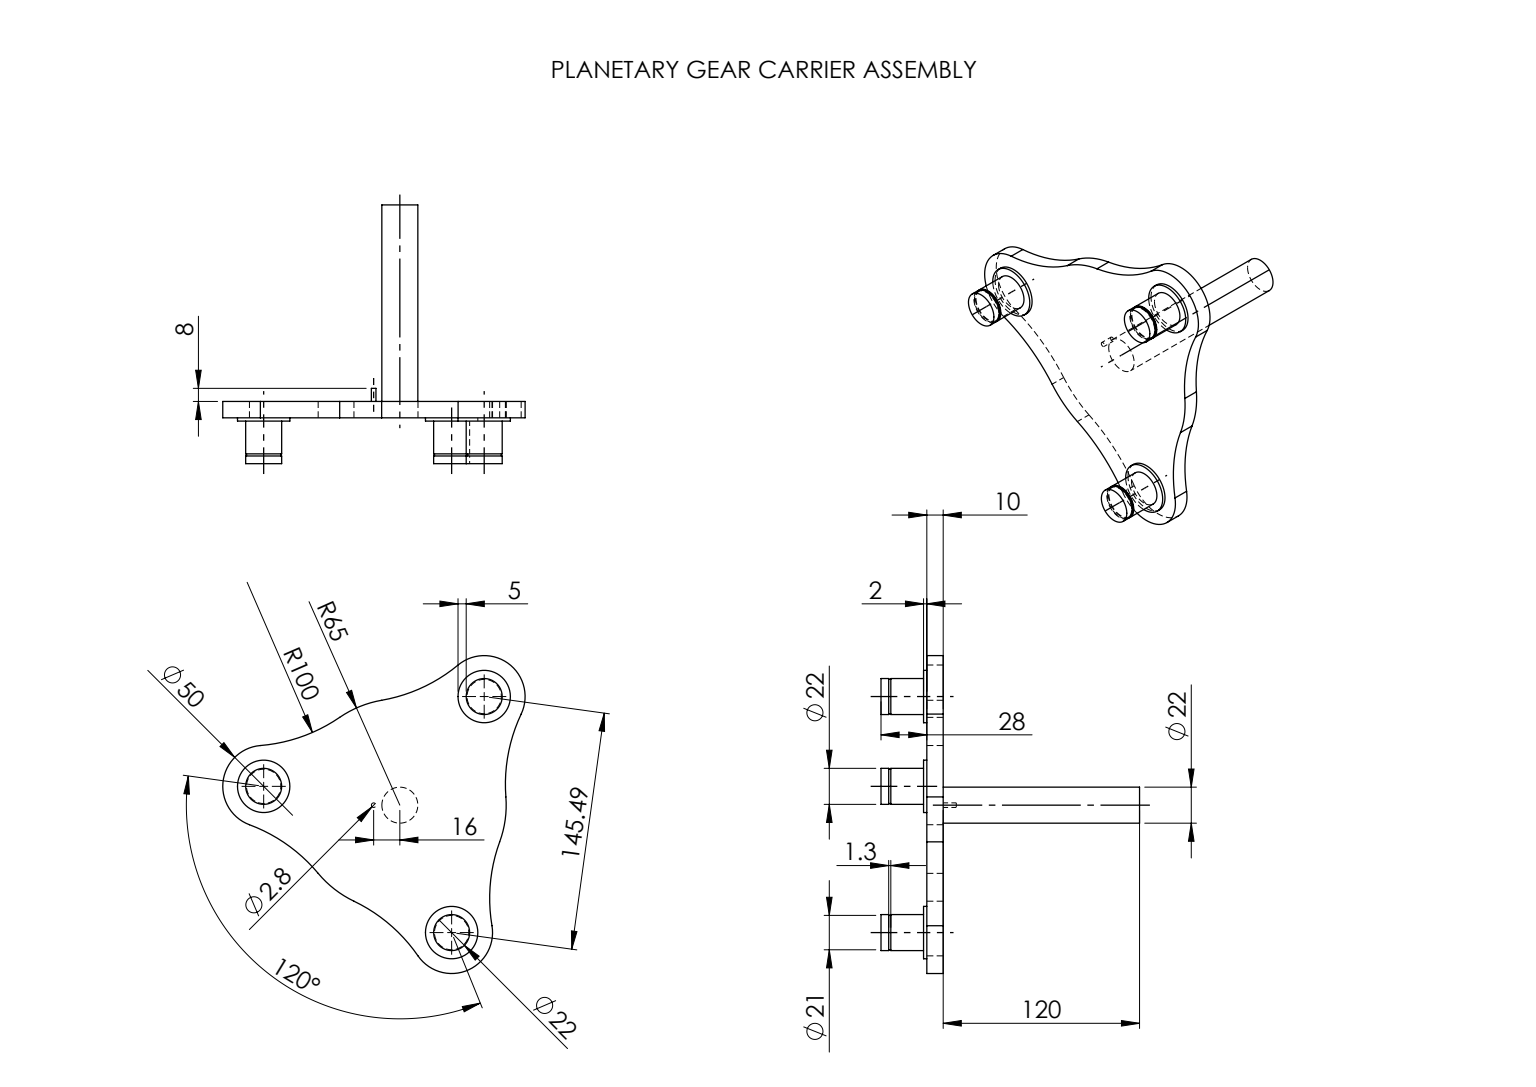
ISO-10303-21;
HEADER;
FILE_DESCRIPTION (('STEP AP214'),
    '1' );
FILE_NAME ('Planetary Gear Carrier Assembly.step',
    '2026-10-08T11:45:07',
    ( '' ),
    ( '' ),
    'SwSTEP 2.0',
    'SolidWorks 2026',
    '' );
FILE_SCHEMA (( 'AUTOMOTIVE_DESIGN' ));
ENDSEC;

DATA;
#3=AXIS2_PLACEMENT_3D ( 'NONE', #17893, #37479, #17456 ) ;
#66=FILL_AREA_STYLE ('',( #17591 ) ) ;
#87=EDGE_CURVE ( 'NONE', #8500, #34172, #3097, .T. ) ;
#134=DIRECTION ( 'NONE',  ( 3.009274222672345096E-17, 1.000000000000000000, -2.455023325076455345E-18 ) ) ;
#185=CARTESIAN_POINT ( 'NONE',  ( 53.30287614962722387, -35.35525454449572180, 69.29271901957299917 ) ) ;
#188=CARTESIAN_POINT ( 'NONE',  ( -36.79328511490363240, -2.055254544495723756, -55.66638716446937707 ) ) ;
#191=EDGE_CURVE ( 'NONE', #37998, #17546, #11534, .T. ) ;
#228=CARTESIAN_POINT ( 'NONE',  ( -102.9608013043458072, -35.35525454449571470, 14.45886780445738218 ) ) ;
#238=FACE_OUTER_BOUND ( 'NONE', #26879, .T. ) ;
#256=MECHANICAL_DESIGN_GEOMETRIC_PRESENTATION_REPRESENTATION('',(#37909),#12862);
#273=AXIS2_PLACEMENT_3D ( 'NONE', #24892, #15283, #24662 ) ;
#300=VERTEX_POINT ( 'NONE', #27299 ) ;
#303=CIRCLE ( 'NONE', #42788, 24.99999999999998934 ) ;
#329=AXIS2_PLACEMENT_3D ( 'NONE', #17951, #33827, #8078 ) ;
#344=EDGE_CURVE ( 'NONE', #2343, #1360, #19212, .T. ) ;
#479=AXIS2_PLACEMENT_3D ( 'NONE', #32329, #9842, #19919 ) ;
#521=SURFACE_STYLE_USAGE ( .BOTH. , #20426 ) ;
#523=ORIENTED_EDGE ( 'NONE', *, *, #10844, .T. ) ;
#530=ORIENTED_EDGE ( 'NONE', *, *, #40112, .T. ) ;
#578=ORIENTED_EDGE ( 'NONE', *, *, #683, .T. ) ;
#610=PLANE ( 'NONE',  #16963 ) ;
#621=CYLINDRICAL_SURFACE ( 'NONE', #22645, 25.00000000000000000 ) ;
#646=DIRECTION ( 'NONE',  ( 1.000000000000000000, -3.009274222672345096E-17, 0.000000000000000000 ) ) ;
#671=DIRECTION ( 'NONE',  ( 3.009274222672345096E-17, 1.000000000000000000, -2.455023325076455345E-18 ) ) ;
#683=EDGE_CURVE ( 'NONE', #23201, #41689, #21250, .T. ) ;
#687=DIRECTION ( 'NONE',  ( -3.009274222672345096E-17, -1.000000000000000000, 2.455023325076454960E-18 ) ) ;
#704=AXIS2_PLACEMENT_3D ( 'NONE', #17398, #27400, #24586 ) ;
#726=SURFACE_STYLE_FILL_AREA ( #66 ) ;
#736=EDGE_CURVE ( 'NONE', #17655, #25229, #13311, .T. ) ;
#775=EDGE_LOOP ( 'NONE', ( #28851, #2876, #36408, #17562 ) ) ;
#804=ADVANCED_FACE ( 'NONE', ( #17457 ), #4302, .T. ) ;
#861=AXIS2_PLACEMENT_3D ( 'NONE', #29019, #9136, #25758 ) ;
#906=ORIENTED_EDGE ( 'NONE', *, *, #34748, .T. ) ;
#938=CARTESIAN_POINT ( 'NONE',  ( 56.05503971749756431, -12.05525454449572464, 8.006123197671259462 ) ) ;
#972=AXIS2_PLACEMENT_3D ( 'NONE', #2544, #29205, #40272 ) ;
#982=EDGE_CURVE ( 'NONE', #41341, #19395, #11317, .T. ) ;
#1003=CARTESIAN_POINT ( 'NONE',  ( 32.30287614962725229, -35.35525454449572180, 69.29271901957299917 ) ) ;
#1019=FILL_AREA_STYLE ('',( #24212 ) ) ;
#1024=DIRECTION ( 'NONE',  ( -1.058513553088275437E-16, -1.000000000000000000, 8.813324511995299047E-17 ) ) ;
#1048=ORIENTED_EDGE ( 'NONE', *, *, #15189, .T. ) ;
#1054=CARTESIAN_POINT ( 'NONE',  ( 26.85238513915532721, -2.055254544495723756, 88.54322126041917329 ) ) ;
#1055=CARTESIAN_POINT ( 'NONE',  ( 42.80287614962790599, -14.05525454449571932, 69.29271901957253021 ) ) ;
#1072=VERTEX_POINT ( 'NONE', #41383 ) ;
#1089=DIRECTION ( 'NONE',  ( 1.000000000000000000, 0.000000000000000000, 0.000000000000000000 ) ) ;
#1168=CYLINDRICAL_SURFACE ( 'NONE', #20654, 11.00000000000023448 ) ;
#1182=CYLINDRICAL_SURFACE ( 'NONE', #32194, 15.99999999999998579 ) ;
#1193=CIRCLE ( 'NONE', #25630, 10.99999999999999822 ) ;
#1295=DIRECTION ( 'NONE',  ( 1.000000000000000000, -3.035766082959412415E-17, 0.000000000000000000 ) ) ;
#1306=ORIENTED_EDGE ( 'NONE', *, *, #9813, .T. ) ;
#1336=CARTESIAN_POINT ( 'NONE',  ( -91.96080130434573618, -35.35525454449571470, 14.45886780445633946 ) ) ;
#1360=VERTEX_POINT ( 'NONE', #26983 ) ;
#1452=DIRECTION ( 'NONE',  ( 3.009274222672345096E-17, 1.000000000000000000, -2.455023325076455345E-18 ) ) ;
#1462=DIRECTION ( 'NONE',  ( 1.000000000000000000, 0.000000000000000000, 0.000000000000000000 ) ) ;
#1493=AXIS2_PLACEMENT_3D ( 'NONE', #14709, #28451, #34754 ) ;
#1543=FACE_BOUND ( 'NONE', #40820, .T. ) ;
#1576=CARTESIAN_POINT ( 'NONE',  ( -91.96080130434580724, -40.05525454449572464, 14.45886780445738218 ) ) ;
#1609=ADVANCED_FACE ( 'NONE', ( #26289 ), #5564, .T. ) ;
#1626=VERTEX_POINT ( 'NONE', #16479 ) ;
#1666=AXIS2_PLACEMENT_3D ( 'NONE', #22494, #18373, #5015 ) ;
#1673=CIRCLE ( 'NONE', #5167, 11.00000000000023803 ) ;
#1684=EDGE_CURVE ( 'NONE', #28176, #33446, #6198, .T. ) ;
#1867=CIRCLE ( 'NONE', #3928, 100.0000000000000711 ) ;
#1931=FACE_OUTER_BOUND ( 'NONE', #23917, .T. ) ;
#1953=CARTESIAN_POINT ( 'NONE',  ( -36.94957890273524725, -12.05525454449572109, 165.5452302238048503 ) ) ;
#1984=ORIENTED_EDGE ( 'NONE', *, *, #344, .T. ) ;
#2031=CARTESIAN_POINT ( 'NONE',  ( 56.25020680251638083, -2.055254544495725977, 2.972870684497274762 ) ) ;
#2040=PLANE ( 'NONE',  #10116 ) ;
#2055=AXIS2_PLACEMENT_3D ( 'NONE', #25182, #17558, #31268 ) ;
#2061=ORIENTED_EDGE ( 'NONE', *, *, #36953, .F. ) ;
#2110=EDGE_LOOP ( 'NONE', ( #9573, #14181, #41848, #41209 ) ) ;
#2116=AXIS2_PLACEMENT_3D ( 'NONE', #27626, #8601, #35009 ) ;
#2146=EDGE_CURVE ( 'NONE', #27084, #7972, #303, .T. ) ;
#2242=EDGE_LOOP ( 'NONE', ( #42171, #17699, #25234, #24047 ) ) ;
#2249=DIRECTION ( 'NONE',  ( -1.000000000000000000, 0.000000000000000000, 0.000000000000000000 ) ) ;
#2261=FACE_OUTER_BOUND ( 'NONE', #9210, .T. ) ;
#2275=DIRECTION ( 'NONE',  ( 1.000000000000000000, 0.000000000000000000, 0.000000000000000000 ) ) ;
#2303=CARTESIAN_POINT ( 'NONE',  ( -19.74979319748359430, -2.055254544495722868, 2.972870684497276539 ) ) ;
#2318=ORIENTED_EDGE ( 'NONE', *, *, #36953, .T. ) ;
#2343=VERTEX_POINT ( 'NONE', #38770 ) ;
#2349=CARTESIAN_POINT ( 'NONE',  ( -8.749793197483594298, -2.055254544495723756, 2.972870684497274762 ) ) ;
#2362=AXIS2_PLACEMENT_3D ( 'NONE', #40085, #9789, #35959 ) ;
#2371=DIRECTION ( 'NONE',  ( 3.009274222672345096E-17, 1.000000000000000000, -2.455023325076454960E-18 ) ) ;
#2386=AXIS2_PLACEMENT_3D ( 'NONE', #30735, #14166, #17017 ) ;
#2406=LINE ( 'NONE', #8773, #18968 ) ;
#2408=PRODUCT_DEFINITION ( 'UNKNOWN', '', #17747, #5868 ) ;
#2428=CIRCLE ( 'NONE', #20624, 11.00000000000023803 ) ;
#2450=ORIENTED_EDGE ( 'NONE', *, *, #18500, .T. ) ;
#2489=ORIENTED_EDGE ( 'NONE', *, *, #34849, .T. ) ;
#2544=CARTESIAN_POINT ( 'NONE',  ( -24.74979319748359785, -2.055254544495722868, 2.972870684497277427 ) ) ;
#2562=CYLINDRICAL_SURFACE ( 'NONE', #12309, 10.99999999999998934 ) ;
#2586=VERTEX_POINT ( 'NONE', #26765 ) ;
#2631=ORIENTED_EDGE ( 'NONE', *, *, #21746, .T. ) ;
#2710=VERTEX_POINT ( 'NONE', #34374 ) ;
#2728=CARTESIAN_POINT ( 'NONE',  ( -80.96080130434580724, -34.05525454449571043, 14.45886780445738395 ) ) ;
#2746=DIRECTION ( 'NONE',  ( -3.009274222672345096E-17, -1.000000000000000000, 2.455023325076455345E-18 ) ) ;
#2762=DIRECTION ( 'NONE',  ( -1.058513553088275437E-16, -1.000000000000000000, 8.813324511995299047E-17 ) ) ;
#2772=EDGE_CURVE ( 'NONE', #25229, #31096, #24877, .T. ) ;
#2872=AXIS2_PLACEMENT_3D ( 'NONE', #31527, #24580, #7523 ) ;
#2876=ORIENTED_EDGE ( 'NONE', *, *, #26728, .T. ) ;
#2898=EDGE_CURVE ( 'NONE', #24559, #19290, #15079, .T. ) ;
#2899=AXIS2_PLACEMENT_3D ( 'NONE', #35121, #37961, #5463 ) ;
#2902=CARTESIAN_POINT ( 'NONE',  ( -80.96080130434580724, -14.05525454449571043, 14.45886780445738395 ) ) ;
#2919=ORIENTED_EDGE ( 'NONE', *, *, #4989, .T. ) ;
#2934=FACE_OUTER_BOUND ( 'NONE', #37750, .T. ) ;
#2987=VERTEX_POINT ( 'NONE', #2902 ) ;
#3055=EDGE_LOOP ( 'NONE', ( #39156, #19434 ) ) ;
#3085=PLANE ( 'NONE',  #20630 ) ;
#3091=VERTEX_POINT ( 'NONE', #36947 ) ;
#3097=CIRCLE ( 'NONE', #15714, 10.99999999999998934 ) ;
#3142=ORIENTED_EDGE ( 'NONE', *, *, #31170, .T. ) ;
#3155=DIRECTION ( 'NONE',  ( -3.009274222672345096E-17, -1.000000000000000000, 2.455023325076454960E-18 ) ) ;
#3191=DIRECTION ( 'NONE',  ( 3.009274222672345096E-17, 1.000000000000000000, -2.455023325076455345E-18 ) ) ;
#3212=FACE_BOUND ( 'NONE', #31827, .T. ) ;
#3262=VECTOR ( 'NONE', #4727, 1000.000000000000000 ) ;
#3286=AXIS2_PLACEMENT_3D ( 'NONE', #23435, #16453, #43031 ) ;
#3299=CIRCLE ( 'NONE', #4699, 11.00000000000023448 ) ;
#3308=APPLICATION_CONTEXT ( 'automotive_design' ) ;
#3319=DIRECTION ( 'NONE',  ( 3.009274222672345096E-17, 1.000000000000000000, -2.455023325076455345E-18 ) ) ;
#3368=ORIENTED_EDGE ( 'NONE', *, *, #14557, .F. ) ;
#3390=AXIS2_PLACEMENT_3D ( 'NONE', #15975, #32107, #19470 ) ;
#3419=CARTESIAN_POINT ( 'NONE',  ( -26.14979319748359643, 5.944745455504278020, 2.972870684497277427 ) ) ;
#3444=( NAMED_UNIT ( * ) SI_UNIT ( $, .STERADIAN. ) SOLID_ANGLE_UNIT ( ) );
#3487=DIRECTION ( 'NONE',  ( -3.009274222672345096E-17, -1.000000000000000000, 2.455023325076454960E-18 ) ) ;
#3534=ORIENTED_EDGE ( 'NONE', *, *, #2146, .F. ) ;
#3555=EDGE_CURVE ( 'NONE', #17655, #26722, #40066, .T. ) ;
#3600=EDGE_CURVE ( 'NONE', #11582, #42604, #23400, .T. ) ;
#3646=DIRECTION ( 'NONE',  ( -1.058513553088275437E-16, -1.000000000000000000, 8.813324511995299047E-17 ) ) ;
#3692=VECTOR ( 'NONE', #37529, 1000.000000000000000 ) ;
#3720=ORIENTED_EDGE ( 'NONE', *, *, #12746, .T. ) ;
#3852=CARTESIAN_POINT ( 'NONE',  ( 0.000000000000000000, 0.000000000000000000, 0.000000000000000000 ) ) ;
#3890=DIRECTION ( 'NONE',  ( -3.009274222672345096E-17, -1.000000000000000000, 2.455023325076454960E-18 ) ) ;
#3898=DIRECTION ( 'NONE',  ( 1.000000000000000000, 0.000000000000000000, 0.000000000000000000 ) ) ;
#3906=EDGE_CURVE ( 'NONE', #6921, #3091, #31737, .T. ) ;
#3928=AXIS2_PLACEMENT_3D ( 'NONE', #1953, #22073, #21653 ) ;
#3933=VECTOR ( 'NONE', #13203, 1000.000000000000000 ) ;
#3936=EDGE_CURVE ( 'NONE', #300, #8500, #22518, .T. ) ;
#3948=VECTOR ( 'NONE', #39099, 1000.000000000000000 ) ;
#3962=ORIENTED_EDGE ( 'NONE', *, *, #5095, .T. ) ;
#3966=AXIS2_PLACEMENT_3D ( 'NONE', #25819, #19275, #32754 ) ;
#3968=CARTESIAN_POINT ( 'NONE',  ( -102.9608013043458072, -40.05525454449572464, 14.45886780445738218 ) ) ;
#4002=DIRECTION ( 'NONE',  ( -1.000000000000000000, 1.084202172485505420E-16, 0.000000000000000000 ) ) ;
#4012=EDGE_CURVE ( 'NONE', #18529, #8193, #11564, .T. ) ;
#4021=ORIENTED_EDGE ( 'NONE', *, *, #14218, .F. ) ;
#4059=LINE ( 'NONE', #24409, #4659 ) ;
#4082=EDGE_CURVE ( 'NONE', #42446, #3091, #42022, .T. ) ;
#4085=DIRECTION ( 'NONE',  ( -1.000000000000000000, 0.000000000000000000, 0.000000000000000000 ) ) ;
#4116=EDGE_CURVE ( 'NONE', #4270, #2710, #25536, .T. ) ;
#4159=EDGE_CURVE ( 'NONE', #19198, #23201, #33152, .T. ) ;
#4169=VERTEX_POINT ( 'NONE', #10441 ) ;
#4257=ORIENTED_EDGE ( 'NONE', *, *, #42315, .F. ) ;
#4270=VERTEX_POINT ( 'NONE', #28654 ) ;
#4278=ORIENTED_EDGE ( 'NONE', *, *, #5722, .F. ) ;
#4293=ADVANCED_FACE ( 'NONE', ( #22133, #38234 ), #15153, .F. ) ;
#4302=CYLINDRICAL_SURFACE ( 'NONE', #2386, 64.99999999999997158 ) ;
#4340=DIRECTION ( 'NONE',  ( -3.009274222672345096E-17, -1.000000000000000000, 2.455023325076455345E-18 ) ) ;
#4359=DIRECTION ( 'NONE',  ( -1.000000000000000000, 0.000000000000000000, 0.000000000000000000 ) ) ;
#4445=ORIENTED_EDGE ( 'NONE', *, *, #23810, .F. ) ;
#4470=SHAPE_REPRESENTATION_RELATIONSHIP ( 'NONE' , 'NONE' ,  #10434, #29166 ) ;
#4495=DIRECTION ( 'NONE',  ( 2.731800627175558911E-17, 1.000000000000000000, -3.170996607629411740E-18 ) ) ;
#4504=AXIS2_PLACEMENT_3D ( 'NONE', #32846, #33283, #16286 ) ;
#4510=DIRECTION ( 'NONE',  ( -3.009274222672345712E-17, -1.000000000000000000, 2.455023325076455345E-18 ) ) ;
#4512=( NAMED_UNIT ( * ) SI_UNIT ( $, .STERADIAN. ) SOLID_ANGLE_UNIT ( ) );
#4543=AXIS2_PLACEMENT_3D ( 'NONE', #43182, #14019, #36672 ) ;
#4544=DIRECTION ( 'NONE',  ( -3.009274222672345096E-17, -1.000000000000000000, 2.455023325076455345E-18 ) ) ;
#4546=CARTESIAN_POINT ( 'NONE',  ( 42.80287614962796994, -2.055254544495723756, 69.29271901957280022 ) ) ;
#4608=CYLINDRICAL_SURFACE ( 'NONE', #15601, 10.49999999999999467 ) ;
#4618=DIRECTION ( 'NONE',  ( 1.000000000000000000, -3.469446951953615421E-17, 0.000000000000000000 ) ) ;
#4644=CIRCLE ( 'NONE', #25586, 100.0000000000000000 ) ;
#4645=DIRECTION ( 'NONE',  ( -1.000000000000000000, 1.084202172485505420E-16, 0.000000000000000000 ) ) ;
#4655=ORIENTED_EDGE ( 'NONE', *, *, #2898, .F. ) ;
#4659=VECTOR ( 'NONE', #14353, 1000.000000000000000 ) ;
#4675=FACE_OUTER_BOUND ( 'NONE', #35556, .T. ) ;
#4688=AXIS2_PLACEMENT_3D ( 'NONE', #26736, #23915, #36969 ) ;
#4699=AXIS2_PLACEMENT_3D ( 'NONE', #10313, #23225, #7236 ) ;
#4705=VERTEX_POINT ( 'NONE', #9098 ) ;
#4727=DIRECTION ( 'NONE',  ( -3.009274222672345096E-17, -1.000000000000000000, 2.455023325076454960E-18 ) ) ;
#4785=DIRECTION ( 'NONE',  ( 1.000000000000000000, -3.469446951953611107E-17, 0.000000000000000000 ) ) ;
#4826=DIRECTION ( 'NONE',  ( 1.058513553088275437E-16, 1.000000000000000000, -8.813324511995299047E-17 ) ) ;
#4836=DIRECTION ( 'NONE',  ( -1.000000000000000000, 0.000000000000000000, 0.000000000000000000 ) ) ;
#4847=CARTESIAN_POINT ( 'NONE',  ( -102.0670434220619427, -12.05525454449572109, 139.0496534599708980 ) ) ;
#4960=CIRCLE ( 'NONE', #11235, 24.99999999999998934 ) ;
#4967=ORIENTED_EDGE ( 'NONE', *, *, #5545, .T. ) ;
#4989=EDGE_CURVE ( 'NONE', #41689, #18808, #4960, .T. ) ;
#5015=DIRECTION ( 'NONE',  ( -1.000000000000000000, 2.668805347656627603E-17, 0.000000000000000000 ) ) ;
#5023=VECTOR ( 'NONE', #21662, 1000.000000000000000 ) ;
#5026=CYLINDRICAL_SURFACE ( 'NONE', #2899, 16.00000000000023448 ) ;
#5037=DIRECTION ( 'NONE',  ( -1.000000000000000000, 0.000000000000000000, 0.000000000000000000 ) ) ;
#5072=CARTESIAN_POINT ( 'NONE',  ( 22.90854556226730310, -35.35525454449573601, -74.83297477053802993 ) ) ;
#5094=DIRECTION ( 'NONE',  ( -1.000000000000000000, 0.000000000000000000, 0.000000000000000000 ) ) ;
#5095=EDGE_CURVE ( 'NONE', #42446, #30653, #33512, .T. ) ;
#5101=FACE_BOUND ( 'NONE', #19325, .T. ) ;
#5115=ADVANCED_FACE ( 'NONE', ( #2261 ), #42190, .F. ) ;
#5143=DIRECTION ( 'NONE',  ( -3.009274222672345096E-17, -1.000000000000000000, 2.455023325076455345E-18 ) ) ;
#5150=VERTEX_POINT ( 'NONE', #12349 ) ;
#5154=DIRECTION ( 'NONE',  ( -1.000000000000000000, 1.577021341797098793E-16, 0.000000000000000000 ) ) ;
#5165=LINE ( 'NONE', #38531, #21399 ) ;
#5167=AXIS2_PLACEMENT_3D ( 'NONE', #12668, #42725, #6310 ) ;
#5180=DIRECTION ( 'NONE',  ( -3.009274222672345096E-17, -1.000000000000000000, 2.455023325076454960E-18 ) ) ;
#5185=ADVANCED_FACE ( 'NONE', ( #19547 ), #39339, .F. ) ;
#5193=DIRECTION ( 'NONE',  ( 1.000000000000000000, -3.469446951953614189E-17, 0.000000000000000000 ) ) ;
#5255=VECTOR ( 'NONE', #29258, 1000.000000000000000 ) ;
#5327=DIRECTION ( 'NONE',  ( 1.000000000000000000, 0.000000000000000000, 0.000000000000000000 ) ) ;
#5343=CYLINDRICAL_SURFACE ( 'NONE', #5646, 10.99999999999999645 ) ;
#5371=DIRECTION ( 'NONE',  ( -1.058513553088275437E-16, -1.000000000000000000, 8.813324511995299047E-17 ) ) ;
#5388=DIRECTION ( 'NONE',  ( -1.058513553088275437E-16, -1.000000000000000000, 8.813324511995299047E-17 ) ) ;
#5394=AXIS2_PLACEMENT_3D ( 'NONE', #15186, #24574, #5327 ) ;
#5397=DIRECTION ( 'NONE',  ( 3.009274222672345096E-17, 1.000000000000000000, -2.455023325076454960E-18 ) ) ;
#5441=ORIENTED_EDGE ( 'NONE', *, *, #32084, .T. ) ;
#5463=DIRECTION ( 'NONE',  ( 1.000000000000000000, 0.000000000000000000, 0.000000000000000000 ) ) ;
#5482=DIRECTION ( 'NONE',  ( 2.932542530036133930E-17, 1.000000000000000000, -5.216001792149171863E-18 ) ) ;
#5515=LINE ( 'NONE', #25199, #25032 ) ;
#5545=EDGE_CURVE ( 'NONE', #28510, #24559, #28465, .T. ) ;
#5564=CYLINDRICAL_SURFACE ( 'NONE', #32515, 15.99999999999999289 ) ;
#5601=EDGE_CURVE ( 'NONE', #23828, #27222, #5515, .T. ) ;
#5624=EDGE_CURVE ( 'NONE', #8001, #13563, #38204, .T. ) ;
#5627=DIRECTION ( 'NONE',  ( -1.000000000000000000, 1.058513553088275437E-16, 0.000000000000000000 ) ) ;
#5646=AXIS2_PLACEMENT_3D ( 'NONE', #9686, #36068, #2249 ) ;
#5684=CARTESIAN_POINT ( 'NONE',  ( 22.90854556226710415, -14.05525454449572997, -74.83297477053821467 ) ) ;
#5695=ORIENTED_EDGE ( 'NONE', *, *, #8889, .T. ) ;
#5722=EDGE_CURVE ( 'NONE', #11152, #9805, #41632, .T. ) ;
#5760=CIRCLE ( 'NONE', #38489, 10.49999999999998934 ) ;
#5768=DIRECTION ( 'NONE',  ( 1.000000000000000000, -3.035766082959414264E-17, 0.000000000000000000 ) ) ;
#5807=ADVANCED_FACE ( 'NONE', ( #28179 ), #11597, .T. ) ;
#5867=CARTESIAN_POINT ( 'NONE',  ( -58.65872368235312706, -2.055254544495720648, -38.66963954070958209 ) ) ;
#5868=PRODUCT_DEFINITION_CONTEXT ( 'detailed design', #3308, 'design' ) ;
#5879=CARTESIAN_POINT ( 'NONE',  ( -24.74979319748359785, 5.944745455504278020, 2.972870684497277427 ) ) ;
#5949=CARTESIAN_POINT ( 'NONE',  ( 56.25020680251638083, -12.05525454449572642, 2.972870684497274762 ) ) ;
#5968=ORIENTED_EDGE ( 'NONE', *, *, #21175, .T. ) ;
#6015=ORIENTED_EDGE ( 'NONE', *, *, #42762, .T. ) ;
#6031=EDGE_LOOP ( 'NONE', ( #27869, #35477, #16575, #38468 ) ) ;
#6088=PLANE ( 'NONE',  #31849 ) ;
#6133=DIRECTION ( 'NONE',  ( -3.009274222672345096E-17, -1.000000000000000000, 2.455023325076454960E-18 ) ) ;
#6160=EDGE_CURVE ( 'NONE', #39731, #1072, #21699, .T. ) ;
#6198=LINE ( 'NONE', #19544, #3933 ) ;
#6277=ORIENTED_EDGE ( 'NONE', *, *, #37983, .F. ) ;
#6283=VERTEX_POINT ( 'NONE', #29904 ) ;
#6301=CARTESIAN_POINT ( 'NONE',  ( -91.96080130434580724, -40.05525454449572464, 14.45886780445738218 ) ) ;
#6310=DIRECTION ( 'NONE',  ( 1.000000000000000000, 0.000000000000000000, 0.000000000000000000 ) ) ;
#6352=CIRCLE ( 'NONE', #40476, 15.99999999999998934 ) ;
#6357=DIRECTION ( 'NONE',  ( 1.000000000000000000, -3.469446951953614189E-17, 0.000000000000000000 ) ) ;
#6360=AXIS2_PLACEMENT_3D ( 'NONE', #6405, #12555, #16478 ) ;
#6391=ORIENTED_EDGE ( 'NONE', *, *, #24742, .T. ) ;
#6401=CYLINDRICAL_SURFACE ( 'NONE', #9809, 10.49999999999998934 ) ;
#6402=PRODUCT_DEFINITION_SHAPE ( 'NONE', 'NONE',  #2408 ) ;
#6405=CARTESIAN_POINT ( 'NONE',  ( 22.90854556226722138, -12.05525454449572464, -74.83297477053847047 ) ) ;
#6457=EDGE_LOOP ( 'NONE', ( #24731, #2631, #43148, #11821 ) ) ;
#6465=DIRECTION ( 'NONE',  ( -3.009274222672345096E-17, -1.000000000000000000, 2.455023325076454960E-18 ) ) ;
#6547=ORIENTED_EDGE ( 'NONE', *, *, #5722, .T. ) ;
#6551=ADVANCED_FACE ( 'NONE', ( #12140 ), #32616, .T. ) ;
#6555=ORIENTED_EDGE ( 'NONE', *, *, #4116, .T. ) ;
#6577=AXIS2_PLACEMENT_3D ( 'NONE', #7725, #18042, #31079 ) ;
#6596=ORIENTED_EDGE ( 'NONE', *, *, #42956, .T. ) ;
#6600=LINE ( 'NONE', #3968, #32014 ) ;
#6606=EDGE_CURVE ( 'NONE', #2710, #4270, #13019, .T. ) ;
#6610=ORIENTED_EDGE ( 'NONE', *, *, #2772, .F. ) ;
#6629=DIRECTION ( 'NONE',  ( -1.000000000000000000, 3.469446951953614189E-17, 0.000000000000000000 ) ) ;
#6683=EDGE_CURVE ( 'NONE', #12272, #25229, #4644, .T. ) ;
#6692=ORIENTED_EDGE ( 'NONE', *, *, #15852, .F. ) ;
#6712=CIRCLE ( 'NONE', #19996, 10.99999999999998934 ) ;
#6714=CARTESIAN_POINT ( 'NONE',  ( -75.96080130434582145, -12.05525454449571043, 14.45886780445738218 ) ) ;
#6727=DIRECTION ( 'NONE',  ( 3.009274222672345096E-17, 1.000000000000000000, -2.455023325076454960E-18 ) ) ;
#6813=LINE ( 'NONE', #15802, #29424 ) ;
#6816=VERTEX_POINT ( 'NONE', #11016 ) ;
#6832=DIRECTION ( 'NONE',  ( -1.000000000000000000, 0.000000000000000000, 0.000000000000000000 ) ) ;
#6853=DIRECTION ( 'NONE',  ( -1.000000000000000000, 0.000000000000000000, 0.000000000000000000 ) ) ;
#6885=DIRECTION ( 'NONE',  ( -3.009274222672345096E-17, -1.000000000000000000, 2.455023325076454960E-18 ) ) ;
#6891=ORIENTED_EDGE ( 'NONE', *, *, #6606, .F. ) ;
#6921=VERTEX_POINT ( 'NONE', #15378 ) ;
#6935=ORIENTED_EDGE ( 'NONE', *, *, #39888, .F. ) ;
#6954=DIRECTION ( 'NONE',  ( 3.009274222672345096E-17, 1.000000000000000000, -2.455023325076454960E-18 ) ) ;
#6974=CIRCLE ( 'NONE', #20263, 10.49999999999999467 ) ;
#6978=DIRECTION ( 'NONE',  ( 3.009274222672345096E-17, 1.000000000000000000, -2.455023325076454960E-18 ) ) ;
#7027=FACE_OUTER_BOUND ( 'NONE', #6031, .T. ) ;
#7080=EDGE_CURVE ( 'NONE', #5150, #12532, #36252, .T. ) ;
#7091=FACE_OUTER_BOUND ( 'NONE', #16629, .T. ) ;
#7103=EDGE_CURVE ( 'NONE', #4270, #4705, #13587, .T. ) ;
#7107=ORIENTED_EDGE ( 'NONE', *, *, #32284, .T. ) ;
#7116=CARTESIAN_POINT ( 'NONE',  ( 146.1418929693599580, -2.055254544495727309, -53.89157828313137344 ) ) ;
#7144=EDGE_LOOP ( 'NONE', ( #16694, #32181 ) ) ;
#7149=CARTESIAN_POINT ( 'NONE',  ( 42.80287614962790599, -34.05525454449571754, 69.29271901957253021 ) ) ;
#7179=CARTESIAN_POINT ( 'NONE',  ( 52.26814377733353467, -2.055254544495723756, -19.42827587850796434 ) ) ;
#7215=AXIS2_PLACEMENT_3D ( 'NONE', #14897, #31025, #14684 ) ;
#7236=DIRECTION ( 'NONE',  ( -1.000000000000000000, 1.577021341797063787E-16, 0.000000000000000000 ) ) ;
#7237=CIRCLE ( 'NONE', #36504, 10.99999999999998934 ) ;
#7242=ORIENTED_EDGE ( 'NONE', *, *, #3906, .F. ) ;
#7394=AXIS2_PLACEMENT_3D ( 'NONE', #5072, #9201, #35393 ) ;
#7416=EDGE_LOOP ( 'NONE', ( #18453, #8451 ) ) ;
#7430=DIRECTION ( 'NONE',  ( -3.009274222672345096E-17, -1.000000000000000000, 2.455023325076454960E-18 ) ) ;
#7451=CARTESIAN_POINT ( 'NONE',  ( 22.90854556226710415, -40.05525454449572464, -74.83297477053821467 ) ) ;
#7457=DIRECTION ( 'NONE',  ( -3.009274222672345096E-17, -1.000000000000000000, 2.455023325076455345E-18 ) ) ;
#7515=DIRECTION ( 'NONE',  ( 2.932542530036133930E-17, 1.000000000000000000, -5.216001792149171863E-18 ) ) ;
#7523=DIRECTION ( 'NONE',  ( 1.000000000000000000, 0.000000000000000000, 0.000000000000000000 ) ) ;
#7567=EDGE_CURVE ( 'NONE', #16411, #23201, #33380, .T. ) ;
#7589=PRESENTATION_STYLE_ASSIGNMENT (( #37474 ) ) ;
#7644=EDGE_LOOP ( 'NONE', ( #25541, #31101, #16059, #2919 ) ) ;
#7646=CYLINDRICAL_SURFACE ( 'NONE', #27613, 10.99999999999999645 ) ;
#7666=AXIS2_PLACEMENT_3D ( 'NONE', #24675, #18797, #34673 ) ;
#7725=CARTESIAN_POINT ( 'NONE',  ( -91.96080130434573618, -35.35525454449571470, 14.45886780445633946 ) ) ;
#7740=FACE_OUTER_BOUND ( 'NONE', #13614, .T. ) ;
#7834=DIRECTION ( 'NONE',  ( -3.009274222672345096E-17, -1.000000000000000000, 2.455023325076454960E-18 ) ) ;
#7906=CARTESIAN_POINT ( 'NONE',  ( -91.96080130434580724, -35.35525454449571470, 14.45886780445738218 ) ) ;
#7924=VECTOR ( 'NONE', #10119, 1000.000000000000000 ) ;
#7933=ORIENTED_EDGE ( 'NONE', *, *, #23388, .T. ) ;
#7942=CARTESIAN_POINT ( 'NONE',  ( -45.51113419504475388, -12.05525454449572109, 56.57887602028989704 ) ) ;
#7951=CARTESIAN_POINT ( 'NONE',  ( -91.96080130434580724, -12.05525454449571043, 14.45886780445738218 ) ) ;
#7963=CARTESIAN_POINT ( 'NONE',  ( 42.80287614962790599, -35.35525454449572180, 69.29271901957253021 ) ) ;
#7972=VERTEX_POINT ( 'NONE', #39855 ) ;
#7987=CYLINDRICAL_SURFACE ( 'NONE', #15209, 10.99999999999998934 ) ;
#8001=VERTEX_POINT ( 'NONE', #40716 ) ;
#8057=ORIENTED_EDGE ( 'NONE', *, *, #17258, .F. ) ;
#8071=AXIS2_PLACEMENT_3D ( 'NONE', #16136, #11628, #21900 ) ;
#8078=DIRECTION ( 'NONE',  ( -1.000000000000000000, 0.000000000000000000, 0.000000000000000000 ) ) ;
#8115=CYLINDRICAL_SURFACE ( 'NONE', #8914, 16.00000000000023448 ) ;
#8116=ORIENTED_EDGE ( 'NONE', *, *, #5624, .F. ) ;
#8137=FACE_OUTER_BOUND ( 'NONE', #2110, .T. ) ;
#8165=CARTESIAN_POINT ( 'NONE',  ( 11.90854556226686789, -34.05525454449573175, -74.83297477053821467 ) ) ;
#8188=DIRECTION ( 'NONE',  ( 1.000000000000000000, 0.000000000000000000, 0.000000000000000000 ) ) ;
#8193=VERTEX_POINT ( 'NONE', #37882 ) ;
#8227=VECTOR ( 'NONE', #7515, 1000.000000000000000 ) ;
#8302=CARTESIAN_POINT ( 'NONE',  ( 65.39325745242679488, -2.055254544495723756, 58.58409293616905700 ) ) ;
#8313=ORIENTED_EDGE ( 'NONE', *, *, #19639, .T. ) ;
#8320=EDGE_CURVE ( 'NONE', #17546, #37998, #17564, .T. ) ;
#8372=CARTESIAN_POINT ( 'NONE',  ( -24.74979319748359785, 5.944745455504278020, 2.972870684497277427 ) ) ;
#8380=DIRECTION ( 'NONE',  ( 1.000000000000000000, -1.058513553088275437E-16, 0.000000000000000000 ) ) ;
#8407=DIRECTION ( 'NONE',  ( 1.000000000000000000, 0.000000000000000000, 0.000000000000000000 ) ) ;
#8424=CIRCLE ( 'NONE', #3, 16.00000000000023448 ) ;
#8437=VECTOR ( 'NONE', #13161, 1000.000000000000000 ) ;
#8451=ORIENTED_EDGE ( 'NONE', *, *, #30150, .F. ) ;
#8500=VERTEX_POINT ( 'NONE', #30666 ) ;
#8508=EDGE_LOOP ( 'NONE', ( #578, #38590, #33423, #40681 ) ) ;
#8543=CYLINDRICAL_SURFACE ( 'NONE', #8071, 100.0000000000000000 ) ;
#8560=CARTESIAN_POINT ( 'NONE',  ( 31.80287614962791665, -34.05525454449571754, 69.29271901957253021 ) ) ;
#8601=DIRECTION ( 'NONE',  ( -3.009274222672345096E-17, -1.000000000000000000, 2.455023325076454960E-18 ) ) ;
#8605=AXIS2_PLACEMENT_3D ( 'NONE', #25733, #2746, #25518 ) ;
#8618=DIRECTION ( 'NONE',  ( 3.009274222672345096E-17, 1.000000000000000000, -2.455023325076454960E-18 ) ) ;
#8656=EDGE_CURVE ( 'NONE', #10648, #300, #21088, .T. ) ;
#8663=DIRECTION ( 'NONE',  ( -3.009274222672345096E-17, -1.000000000000000000, 2.455023325076454960E-18 ) ) ;
#8676=ORIENTED_EDGE ( 'NONE', *, *, #25735, .F. ) ;
#8677=CYLINDRICAL_SURFACE ( 'NONE', #8605, 15.99999999999998579 ) ;
#8686=ADVANCED_FACE ( 'NONE', ( #7740 ), #1182, .T. ) ;
#8690=CIRCLE ( 'NONE', #4504, 10.99999999999999822 ) ;
#8745=DIRECTION ( 'NONE',  ( 1.000000000000000000, 0.000000000000000000, 0.000000000000000000 ) ) ;
#8773=CARTESIAN_POINT ( 'NONE',  ( -58.65872368235312706, -2.055254544495720648, -38.66963954070958209 ) ) ;
#8822=FACE_OUTER_BOUND ( 'NONE', #32539, .T. ) ;
#8889=EDGE_CURVE ( 'NONE', #2710, #42617, #16849, .T. ) ;
#8914=AXIS2_PLACEMENT_3D ( 'NONE', #11624, #28207, #17760 ) ;
#8974=CARTESIAN_POINT ( 'NONE',  ( -75.96080130434582145, -12.05525454449572109, 14.45886780445738218 ) ) ;
#8981=ORIENTED_EDGE ( 'NONE', *, *, #43083, .T. ) ;
#9002=ORIENTED_EDGE ( 'NONE', *, *, #24578, .T. ) ;
#9047=DIRECTION ( 'NONE',  ( -3.009274222672345096E-17, -1.000000000000000000, 2.455023325076455345E-18 ) ) ;
#9063=DIRECTION ( 'NONE',  ( -1.058513553088275437E-16, -1.000000000000000000, 8.813324511995299047E-17 ) ) ;
#9098=CARTESIAN_POINT ( 'NONE',  ( 26.80287614962791309, -14.05525454449571754, 69.29271901957253021 ) ) ;
#9136=DIRECTION ( 'NONE',  ( -3.009274222672345096E-17, -1.000000000000000000, 2.455023325076454960E-18 ) ) ;
#9159=LINE ( 'NONE', #16373, #27450 ) ;
#9201=DIRECTION ( 'NONE',  ( -1.058513553088275437E-16, -1.000000000000000000, 8.813324511995299047E-17 ) ) ;
#9210=EDGE_LOOP ( 'NONE', ( #25750, #28064, #21092, #17412 ) ) ;
#9213=VERTEX_POINT ( 'NONE', #35528 ) ;
#9234=CARTESIAN_POINT ( 'NONE',  ( 67.80287614962797704, -2.055254544495724645, 69.29271901957280022 ) ) ;
#9265=CARTESIAN_POINT ( 'NONE',  ( -91.96080130434580724, -34.05525454449571043, 14.45886780445738218 ) ) ;
#9331=FACE_BOUND ( 'NONE', #35580, .T. ) ;
#9336=EDGE_CURVE ( 'NONE', #41904, #17494, #32925, .T. ) ;
#9355=AXIS2_PLACEMENT_3D ( 'NONE', #38969, #3155, #13251 ) ;
#9356=ORIENTED_EDGE ( 'NONE', *, *, #17580, .F. ) ;
#9364=CIRCLE ( 'NONE', #273, 25.00000000000000000 ) ;
#9369=DIRECTION ( 'NONE',  ( -1.058513553088275437E-16, -1.000000000000000000, 8.813324511995299047E-17 ) ) ;
#9414=DIRECTION ( 'NONE',  ( 1.000000000000000000, 0.000000000000000000, 0.000000000000000000 ) ) ;
#9426=STYLED_ITEM ( 'NONE', ( #33686 ), #27879 ) ;
#9573=ORIENTED_EDGE ( 'NONE', *, *, #42762, .F. ) ;
#9580=DIRECTION ( 'NONE',  ( 1.000000000000000000, 0.000000000000000000, 0.000000000000000000 ) ) ;
#9603=ADVANCED_FACE ( 'NONE', ( #28332 ), #34404, .T. ) ;
#9686=CARTESIAN_POINT ( 'NONE',  ( -91.96080130434580724, -40.05525454449572464, 14.45886780445738218 ) ) ;
#9708=CIRCLE ( 'NONE', #3390, 10.99999999999999645 ) ;
#9769=ADVANCED_FACE ( 'NONE', ( #2934 ), #29183, .T. ) ;
#9789=DIRECTION ( 'NONE',  ( -3.009274222672345096E-17, -1.000000000000000000, 2.455023325076454960E-18 ) ) ;
#9805=VERTEX_POINT ( 'NONE', #38751 ) ;
#9809=AXIS2_PLACEMENT_3D ( 'NONE', #29550, #13199, #16252 ) ;
#9813=EDGE_CURVE ( 'NONE', #34600, #23370, #16075, .T. ) ;
#9821=DIRECTION ( 'NONE',  ( -1.058513553088275437E-16, -1.000000000000000000, 8.813324511995299047E-17 ) ) ;
#9842=DIRECTION ( 'NONE',  ( -1.058513553088275437E-16, -1.000000000000000000, 8.813324511995299047E-17 ) ) ;
#9848=ORIENTED_EDGE ( 'NONE', *, *, #16957, .F. ) ;
#9874=VERTEX_POINT ( 'NONE', #23926 ) ;
#9881=DIRECTION ( 'NONE',  ( 1.000000000000000000, 0.000000000000000000, 0.000000000000000000 ) ) ;
#9907=CARTESIAN_POINT ( 'NONE',  ( -135.4416936590755540, -12.05525454449572109, -102.7350398871816424 ) ) ;
#9932=CARTESIAN_POINT ( 'NONE',  ( 11.90854556226686789, -40.05525454449572464, -74.83297477053821467 ) ) ;
#9951=ADVANCED_FACE ( 'NONE', ( #7091 ), #30460, .T. ) ;
#9957=ORIENTED_EDGE ( 'NONE', *, *, #34849, .F. ) ;
#9970=VERTEX_POINT ( 'NONE', #40667 ) ;
#9981=ADVANCED_FACE ( 'NONE', ( #20668 ), #33935, .T. ) ;
#10014=CARTESIAN_POINT ( 'NONE',  ( -93.98204972788910538, -2.055254544495720648, 39.37702493556011518 ) ) ;
#10019=AXIS2_PLACEMENT_3D ( 'NONE', #5879, #2371, #32506 ) ;
#10034=EDGE_CURVE ( 'NONE', #18362, #43113, #6974, .T. ) ;
#10050=PLANE ( 'NONE',  #31049 ) ;
#10060=ADVANCED_FACE ( 'NONE', ( #18270 ), #18480, .F. ) ;
#10079=CARTESIAN_POINT ( 'NONE',  ( -91.96080130434580724, -40.05525454449572464, 14.45886780445738218 ) ) ;
#10116=AXIS2_PLACEMENT_3D ( 'NONE', #18902, #25651, #18700 ) ;
#10119=DIRECTION ( 'NONE',  ( -3.009274222672345096E-17, -1.000000000000000000, 2.455023325076454960E-18 ) ) ;
#10208=ADVANCED_FACE ( 'NONE', ( #18914 ), #5343, .T. ) ;
#10213=DIRECTION ( 'NONE',  ( 1.000000000000000000, 0.000000000000000000, 0.000000000000000000 ) ) ;
#10313=CARTESIAN_POINT ( 'NONE',  ( 22.90854556226710415, -14.05525454449572997, -74.83297477053821467 ) ) ;
#10360=DIRECTION ( 'NONE',  ( 1.058513553088275437E-16, 1.000000000000000000, -8.813324511995299047E-17 ) ) ;
#10370=ADVANCED_FACE ( 'NONE', ( #27353 ), #33009, .T. ) ;
#10384=UNCERTAINTY_MEASURE_WITH_UNIT (LENGTH_MEASURE( 1.000000000000000082E-05 ), #23770, 'distance_accuracy_value', 'NONE');
#10399=LINE ( 'NONE', #23732, #21861 ) ;
#10416=CIRCLE ( 'NONE', #12614, 10.49999999999998934 ) ;
#10434=SHAPE_REPRESENTATION ( 'Planetary Gear Carrier Assembly', ( #13552 ), #21242 ) ;
#10441=CARTESIAN_POINT ( 'NONE',  ( -102.9608013043458072, -40.05525454449572464, 14.45886780445738218 ) ) ;
#10619=EDGE_CURVE ( 'NONE', #4705, #42617, #6352, .T. ) ;
#10624=FACE_OUTER_BOUND ( 'NONE', #27357, .T. ) ;
#10648=VERTEX_POINT ( 'NONE', #25387 ) ;
#10665=DIRECTION ( 'NONE',  ( -1.000000000000000000, 1.058513553088275437E-16, 0.000000000000000000 ) ) ;
#10684=ORIENTED_EDGE ( 'NONE', *, *, #27058, .F. ) ;
#10768=CIRCLE ( 'NONE', #21956, 15.99999999999998579 ) ;
#10799=CARTESIAN_POINT ( 'NONE',  ( -81.46080130434573618, -35.35525454449571470, 14.45886780445633946 ) ) ;
#10803=AXIS2_PLACEMENT_3D ( 'NONE', #39705, #16199, #20141 ) ;
#10811=DIRECTION ( 'NONE',  ( -1.000000000000000000, 1.577021341797097807E-16, 0.000000000000000000 ) ) ;
#10844=EDGE_CURVE ( 'NONE', #14319, #19640, #14744, .T. ) ;
#10851=MECHANICAL_DESIGN_GEOMETRIC_PRESENTATION_REPRESENTATION('',(#9426),#42861);
#10871=ADVANCED_FACE ( 'NONE', ( #37898 ), #11762, .T. ) ;
#10884=CARTESIAN_POINT ( 'NONE',  ( 22.90854556226730310, -35.35525454449573601, -74.83297477053802993 ) ) ;
#10898=DIRECTION ( 'NONE',  ( 1.058513553088275437E-16, 1.000000000000000000, -8.813324511995299047E-17 ) ) ;
#10918=LINE ( 'NONE', #33161, #33003 ) ;
#10982=FACE_OUTER_BOUND ( 'NONE', #26734, .T. ) ;
#10991=DIRECTION ( 'NONE',  ( 1.000000000000000000, 0.000000000000000000, 0.000000000000000000 ) ) ;
#11011=AXIS2_PLACEMENT_3D ( 'NONE', #24283, #11375, #1089 ) ;
#11016=CARTESIAN_POINT ( 'NONE',  ( -36.79328511490363240, -2.055254544495723756, -55.66638716446937707 ) ) ;
#11060=CARTESIAN_POINT ( 'NONE',  ( 22.90854556226722138, -12.05525454449572464, -74.83297477053847047 ) ) ;
#11081=ORIENTED_EDGE ( 'NONE', *, *, #17716, .T. ) ;
#11110=CARTESIAN_POINT ( 'NONE',  ( -75.96080130434582145, -14.05525454449571221, 14.45886780445738218 ) ) ;
#11144=CARTESIAN_POINT ( 'NONE',  ( 58.80287614962789888, -12.05525454449571932, 69.29271901957253021 ) ) ;
#11152=VERTEX_POINT ( 'NONE', #38970 ) ;
#11199=DIRECTION ( 'NONE',  ( -1.000000000000000000, 3.009274222672345096E-17, 0.000000000000000000 ) ) ;
#11235=AXIS2_PLACEMENT_3D ( 'NONE', #11060, #21566, #11486 ) ;
#11242=PLANE ( 'NONE',  #15846 ) ;
#11297=ORIENTED_EDGE ( 'NONE', *, *, #15080, .T. ) ;
#11315=FACE_OUTER_BOUND ( 'NONE', #12946, .T. ) ;
#11317=LINE ( 'NONE', #35284, #16615 ) ;
#11375=DIRECTION ( 'NONE',  ( -3.009274222672345096E-17, -1.000000000000000000, 2.455023325076455345E-18 ) ) ;
#11409=DIRECTION ( 'NONE',  ( 3.009274222672345096E-17, 1.000000000000000000, -2.455023325076454960E-18 ) ) ;
#11420=EDGE_CURVE ( 'NONE', #12532, #19198, #6813, .T. ) ;
#11423=DIRECTION ( 'NONE',  ( 3.009274222672345096E-17, 1.000000000000000000, -2.455023325076455345E-18 ) ) ;
#11430=CARTESIAN_POINT ( 'NONE',  ( 53.80287614962789178, -35.35525454449572180, 69.29271901957253021 ) ) ;
#11434=CARTESIAN_POINT ( 'NONE',  ( 11.90854556226686789, -35.35525454449573601, -74.83297477053821467 ) ) ;
#11453=ORIENTED_EDGE ( 'NONE', *, *, #28624, .F. ) ;
#11474=CIRCLE ( 'NONE', #1666, 64.99999999999997158 ) ;
#11486=DIRECTION ( 'NONE',  ( -1.000000000000000000, 0.000000000000000000, 0.000000000000000000 ) ) ;
#11522=EDGE_CURVE ( 'NONE', #2343, #25188, #26896, .T. ) ;
#11529=DIRECTION ( 'NONE',  ( -3.009274222672345096E-17, -1.000000000000000000, 2.455023325076455345E-18 ) ) ;
#11534=CIRCLE ( 'NONE', #10803, 11.00000000000023803 ) ;
#11564=CIRCLE ( 'NONE', #22728, 11.00000000000023448 ) ;
#11578=EDGE_LOOP ( 'NONE', ( #19413, #24882, #6596, #18060 ) ) ;
#11582=VERTEX_POINT ( 'NONE', #228 ) ;
#11588=ORIENTED_EDGE ( 'NONE', *, *, #38643, .F. ) ;
#11597=CYLINDRICAL_SURFACE ( 'NONE', #11011, 1.399999999999998579 ) ;
#11624=CARTESIAN_POINT ( 'NONE',  ( 22.90854556226710415, -12.05525454449572997, -74.83297477053821467 ) ) ;
#11628=DIRECTION ( 'NONE',  ( -3.009274222672345096E-17, -1.000000000000000000, 2.455023325076454960E-18 ) ) ;
#11715=CARTESIAN_POINT ( 'NONE',  ( 22.90854556226730310, -35.35525454449573601, -74.83297477053802993 ) ) ;
#11720=DIRECTION ( 'NONE',  ( -1.000000000000000000, 0.000000000000000000, 0.000000000000000000 ) ) ;
#11762=CYLINDRICAL_SURFACE ( 'NONE', #23836, 15.99999999999999289 ) ;
#11774=AXIS2_PLACEMENT_3D ( 'NONE', #26018, #35795, #9414 ) ;
#11791=AXIS2_PLACEMENT_3D ( 'NONE', #29482, #6978, #17056 ) ;
#11821=ORIENTED_EDGE ( 'NONE', *, *, #28389, .F. ) ;
#11829=CARTESIAN_POINT ( 'NONE',  ( -91.96080130434580724, -14.05525454449570866, 14.45886780445738218 ) ) ;
#11926=EDGE_LOOP ( 'NONE', ( #7933, #17011, #36278, #5441 ) ) ;
#11992=DIRECTION ( 'NONE',  ( -3.009274222672345096E-17, -1.000000000000000000, 2.455023325076454960E-18 ) ) ;
#12094=EDGE_LOOP ( 'NONE', ( #6277, #37035, #29960, #35486 ) ) ;
#12137=EDGE_CURVE ( 'NONE', #300, #10648, #7237, .T. ) ;
#12140=FACE_OUTER_BOUND ( 'NONE', #43036, .T. ) ;
#12150=CARTESIAN_POINT ( 'NONE',  ( 42.80287614962790599, -40.05525454449572464, 69.29271901957253021 ) ) ;
#12165=DIRECTION ( 'NONE',  ( -3.009274222672345096E-17, -1.000000000000000000, 2.455023325076454960E-18 ) ) ;
#12189=DIRECTION ( 'NONE',  ( -1.058513553088275437E-16, -1.000000000000000000, 8.813324511995299047E-17 ) ) ;
#12193=ORIENTED_EDGE ( 'NONE', *, *, #24578, .F. ) ;
#12197=CYLINDRICAL_SURFACE ( 'NONE', #21939, 25.00000000000000000 ) ;
#12246=DIRECTION ( 'NONE',  ( 1.058513553088275437E-16, 1.000000000000000000, -8.813324511995299047E-17 ) ) ;
#12272=VERTEX_POINT ( 'NONE', #20428 ) ;
#12282=DIRECTION ( 'NONE',  ( 3.009274222672345096E-17, 1.000000000000000000, -2.455023325076454960E-18 ) ) ;
#12308=LINE ( 'NONE', #25215, #3948 ) ;
#12309=AXIS2_PLACEMENT_3D ( 'NONE', #16334, #3191, #19421 ) ;
#12349=CARTESIAN_POINT ( 'NONE',  ( 56.05503971749756431, -2.055254544495723756, 8.006123197671259462 ) ) ;
#12357=CIRCLE ( 'NONE', #24935, 10.49999999999998934 ) ;
#12360=CARTESIAN_POINT ( 'NONE',  ( 22.90854556226730310, -35.35525454449573601, -74.83297477053802993 ) ) ;
#12442=ORIENTED_EDGE ( 'NONE', *, *, #38151, .F. ) ;
#12485=EDGE_CURVE ( 'NONE', #38421, #1626, #24770, .T. ) ;
#12494=CARTESIAN_POINT ( 'NONE',  ( 42.80287614962790599, -14.05525454449571932, 69.29271901957253021 ) ) ;
#12513=ORIENTED_EDGE ( 'NONE', *, *, #28624, .T. ) ;
#12532=VERTEX_POINT ( 'NONE', #2031 ) ;
#12555=DIRECTION ( 'NONE',  ( 3.009274222672345096E-17, 1.000000000000000000, -2.455023325076454960E-18 ) ) ;
#12591=ORIENTED_EDGE ( 'NONE', *, *, #3555, .T. ) ;
#12614=AXIS2_PLACEMENT_3D ( 'NONE', #30526, #1024, #33996 ) ;
#12634=FACE_OUTER_BOUND ( 'NONE', #16127, .T. ) ;
#12668=CARTESIAN_POINT ( 'NONE',  ( 22.90854556226710415, -40.05525454449572464, -74.83297477053821467 ) ) ;
#12673=ADVANCED_FACE ( 'NONE', ( #34443 ), #621, .T. ) ;
#12693=ORIENTED_EDGE ( 'NONE', *, *, #42792, .F. ) ;
#12694=DIRECTION ( 'NONE',  ( -3.009274222672345096E-17, -1.000000000000000000, 2.455023325076454960E-18 ) ) ;
#12706=ORIENTED_EDGE ( 'NONE', *, *, #34165, .F. ) ;
#12715=DIRECTION ( 'NONE',  ( 3.009274222672345096E-17, 1.000000000000000000, -2.455023325076455345E-18 ) ) ;
#12737=DIRECTION ( 'NONE',  ( -1.000000000000000000, 0.000000000000000000, 0.000000000000000000 ) ) ;
#12746=EDGE_CURVE ( 'NONE', #42617, #4705, #40708, .T. ) ;
#12768=CARTESIAN_POINT ( 'NONE',  ( -79.93711883401132923, -2.055254544495720648, -145.8806300090334673 ) ) ;
#12777=DIRECTION ( 'NONE',  ( 3.009274222672345096E-17, 1.000000000000000000, -2.455023325076454960E-18 ) ) ;
#12797=DIRECTION ( 'NONE',  ( -1.058513553088275437E-16, -1.000000000000000000, 8.813324511995299047E-17 ) ) ;
#12862=( GEOMETRIC_REPRESENTATION_CONTEXT ( 3 ) GLOBAL_UNCERTAINTY_ASSIGNED_CONTEXT ( ( #21763 ) ) GLOBAL_UNIT_ASSIGNED_CONTEXT ( ( #33766, #17238, #3444 ) ) REPRESENTATION_CONTEXT ( 'NONE', 'WORKASPACE' ) );
#12879=CARTESIAN_POINT ( 'NONE',  ( 42.80287614962796994, -12.05525454449572464, 69.29271901957280022 ) ) ;
#12892=FACE_OUTER_BOUND ( 'NONE', #22229, .T. ) ;
#12896=VECTOR ( 'NONE', #19221, 1000.000000000000000 ) ;
#12926=AXIS2_PLACEMENT_3D ( 'NONE', #35980, #9369, #22725 ) ;
#12946=EDGE_LOOP ( 'NONE', ( #11453, #14481, #17138, #33898 ) ) ;
#12952=DIRECTION ( 'NONE',  ( 1.000000000000000000, 0.000000000000000000, 0.000000000000000000 ) ) ;
#13010=VECTOR ( 'NONE', #40055, 1000.000000000000000 ) ;
#13019=CIRCLE ( 'NONE', #38776, 15.99999999999998934 ) ;
#13092=DIRECTION ( 'NONE',  ( 1.000000000000000000, 0.000000000000000000, 0.000000000000000000 ) ) ;
#13138=ORIENTED_EDGE ( 'NONE', *, *, #14876, .T. ) ;
#13145=PLANE ( 'NONE',  #41491 ) ;
#13161=DIRECTION ( 'NONE',  ( -3.009274222672345096E-17, -1.000000000000000000, 2.455023325076455345E-18 ) ) ;
#13166=ADVANCED_FACE ( 'NONE', ( #9331, #19622 ), #22687, .F. ) ;
#13199=DIRECTION ( 'NONE',  ( 2.731800627175558911E-17, 1.000000000000000000, -3.170996607629411740E-18 ) ) ;
#13203=DIRECTION ( 'NONE',  ( 3.009274222672345096E-17, 1.000000000000000000, -2.455023325076455345E-18 ) ) ;
#13227=DIRECTION ( 'NONE',  ( -3.009274222672345712E-17, -1.000000000000000000, 2.455023325076455345E-18 ) ) ;
#13250=ORIENTED_EDGE ( 'NONE', *, *, #17227, .T. ) ;
#13251=DIRECTION ( 'NONE',  ( 1.000000000000000000, -3.035766082959412415E-17, 0.000000000000000000 ) ) ;
#13288=ORIENTED_EDGE ( 'NONE', *, *, #5624, .T. ) ;
#13311=LINE ( 'NONE', #36179, #12896 ) ;
#13396=DIRECTION ( 'NONE',  ( -1.058513553088275437E-16, -1.000000000000000000, 8.813324511995299047E-17 ) ) ;
#13438=( NAMED_UNIT ( * ) PLANE_ANGLE_UNIT ( ) SI_UNIT ( $, .RADIAN. ) );
#13457=CARTESIAN_POINT ( 'NONE',  ( 42.80287614962723808, -35.35525454449572180, 69.29271901957299917 ) ) ;
#13552=AXIS2_PLACEMENT_3D ( 'NONE', #3852, #14597, #10213 ) ;
#13563=VERTEX_POINT ( 'NONE', #11434 ) ;
#13576=CARTESIAN_POINT ( 'NONE',  ( -91.96080130434580724, -40.05525454449572464, 14.45886780445738218 ) ) ;
#13587=LINE ( 'NONE', #36674, #8437 ) ;
#13614=EDGE_LOOP ( 'NONE', ( #8981, #32037, #17705, #19043 ) ) ;
#13621=EDGE_LOOP ( 'NONE', ( #29673, #21273 ) ) ;
#13700=ORIENTED_EDGE ( 'NONE', *, *, #14633, .F. ) ;
#13752=DIRECTION ( 'NONE',  ( 1.058513553088275437E-16, 1.000000000000000000, -8.813324511995299047E-17 ) ) ;
#13769=CARTESIAN_POINT ( 'NONE',  ( 53.30287614962722387, -34.05525454449571754, 69.29271901957299917 ) ) ;
#13784=AXIS2_PLACEMENT_3D ( 'NONE', #41047, #11409, #11199 ) ;
#13800=CARTESIAN_POINT ( 'NONE',  ( -91.96080130434573618, -34.05525454449571043, 14.45886780445633946 ) ) ;
#13816=DIRECTION ( 'NONE',  ( -3.009274222672345096E-17, -1.000000000000000000, 2.455023325076454960E-18 ) ) ;
#13833=ORIENTED_EDGE ( 'NONE', *, *, #4989, .F. ) ;
#13888=CARTESIAN_POINT ( 'NONE',  ( -91.96080130434580724, -14.05525454449570866, 14.45886780445738218 ) ) ;
#13896=EDGE_CURVE ( 'NONE', #30077, #21731, #25011, .T. ) ;
#14019=DIRECTION ( 'NONE',  ( -1.058513553088275437E-16, -1.000000000000000000, 8.813324511995299047E-17 ) ) ;
#14023=ORIENTED_EDGE ( 'NONE', *, *, #4159, .F. ) ;
#14040=DIRECTION ( 'NONE',  ( 3.009274222672345096E-17, 1.000000000000000000, -2.455023325076454960E-18 ) ) ;
#14089=ADVANCED_FACE ( 'NONE', ( #37338 ), #40592, .T. ) ;
#14163=ORIENTED_EDGE ( 'NONE', *, *, #36153, .T. ) ;
#14166=DIRECTION ( 'NONE',  ( -3.009274222672345096E-17, -1.000000000000000000, 2.455023325076454960E-18 ) ) ;
#14169=ORIENTED_EDGE ( 'NONE', *, *, #7103, .T. ) ;
#14181=ORIENTED_EDGE ( 'NONE', *, *, #16957, .T. ) ;
#14212=ORIENTED_EDGE ( 'NONE', *, *, #5545, .F. ) ;
#14218=EDGE_CURVE ( 'NONE', #34135, #22843, #18648, .T. ) ;
#14250=DIRECTION ( 'NONE',  ( -3.009274222672345096E-17, -1.000000000000000000, 2.455023325076454960E-18 ) ) ;
#14302=ORIENTED_EDGE ( 'NONE', *, *, #32005, .T. ) ;
#14319=VERTEX_POINT ( 'NONE', #38618 ) ;
#14324=EDGE_CURVE ( 'NONE', #30077, #24613, #36693, .T. ) ;
#14330=AXIS2_PLACEMENT_3D ( 'NONE', #16212, #29508, #42776 ) ;
#14353=DIRECTION ( 'NONE',  ( 3.009274222672345096E-17, 1.000000000000000000, -2.455023325076455345E-18 ) ) ;
#14354=ORIENTED_EDGE ( 'NONE', *, *, #12485, .F. ) ;
#14368=AXIS2_PLACEMENT_3D ( 'NONE', #18533, #5397, #18761 ) ;
#14406=FACE_BOUND ( 'NONE', #28309, .T. ) ;
#14438=AXIS2_PLACEMENT_3D ( 'NONE', #8372, #14519, #14952 ) ;
#14481=ORIENTED_EDGE ( 'NONE', *, *, #5095, .F. ) ;
#14519=DIRECTION ( 'NONE',  ( 3.009274222672345096E-17, 1.000000000000000000, -2.455023325076454960E-18 ) ) ;
#14557=EDGE_CURVE ( 'NONE', #9213, #42604, #4059, .T. ) ;
#14578=LINE ( 'NONE', #27882, #3262 ) ;
#14592=CARTESIAN_POINT ( 'NONE',  ( 53.80287614962789178, -34.05525454449571754, 69.29271901957253021 ) ) ;
#14597=DIRECTION ( 'NONE',  ( 0.000000000000000000, 0.000000000000000000, 1.000000000000000000 ) ) ;
#14633=EDGE_CURVE ( 'NONE', #7972, #11152, #14578, .T. ) ;
#14684=DIRECTION ( 'NONE',  ( 1.000000000000000000, 0.000000000000000000, 0.000000000000000000 ) ) ;
#14709=CARTESIAN_POINT ( 'NONE',  ( 22.90854556226710415, -12.05525454449572464, -74.83297477053821467 ) ) ;
#14719=CARTESIAN_POINT ( 'NONE',  ( -23.34979319748359927, -2.055254544495722868, 2.972870684497277427 ) ) ;
#14744=CIRCLE ( 'NONE', #19633, 15.99999999999998579 ) ;
#14799=EDGE_LOOP ( 'NONE', ( #12591, #14302, #19116, #4967, #22410, #7107, #39331, #33392, #15277, #23433, #19643, #20461, #18451, #14163, #6391 ) ) ;
#14876=EDGE_CURVE ( 'NONE', #19395, #27222, #21483, .T. ) ;
#14897=CARTESIAN_POINT ( 'NONE',  ( 22.90854556226730310, -35.35525454449573601, -74.83297477053802993 ) ) ;
#14907=ORIENTED_EDGE ( 'NONE', *, *, #37157, .T. ) ;
#14922=CARTESIAN_POINT ( 'NONE',  ( -93.98204972788910538, -2.055254544495720648, 39.37702493556011518 ) ) ;
#14926=VECTOR ( 'NONE', #34028, 1000.000000000000000 ) ;
#14952=DIRECTION ( 'NONE',  ( -1.000000000000000000, 0.000000000000000000, 0.000000000000000000 ) ) ;
#14953=FACE_OUTER_BOUND ( 'NONE', #20971, .T. ) ;
#14968=CARTESIAN_POINT ( 'NONE',  ( 33.40854556226729954, -35.35525454449573601, -74.83297477053802993 ) ) ;
#15079=CIRCLE ( 'NONE', #39403, 25.00000000000000000 ) ;
#15080=EDGE_CURVE ( 'NONE', #38421, #43113, #34558, .T. ) ;
#15097=LINE ( 'NONE', #8302, #5023 ) ;
#15099=ORIENTED_EDGE ( 'NONE', *, *, #27755, .T. ) ;
#15130=ORIENTED_EDGE ( 'NONE', *, *, #344, .F. ) ;
#15153=PLANE ( 'NONE',  #7394 ) ;
#15157=DIRECTION ( 'NONE',  ( 1.058513553088275437E-16, 1.000000000000000000, -8.813324511995299047E-17 ) ) ;
#15186=CARTESIAN_POINT ( 'NONE',  ( 22.90854556226730310, -34.05525454449573175, -74.83297477053802993 ) ) ;
#15189=EDGE_CURVE ( 'NONE', #1626, #18362, #38047, .T. ) ;
#15209=AXIS2_PLACEMENT_3D ( 'NONE', #40922, #24402, #30906 ) ;
#15216=AXIS2_PLACEMENT_3D ( 'NONE', #40602, #27126, #36692 ) ;
#15242=AXIS2_PLACEMENT_3D ( 'NONE', #41284, #24765, #38021 ) ;
#15277=ORIENTED_EDGE ( 'NONE', *, *, #32217, .T. ) ;
#15283=DIRECTION ( 'NONE',  ( 3.009274222672345096E-17, 1.000000000000000000, -2.455023325076454960E-18 ) ) ;
#15315=EDGE_CURVE ( 'NONE', #9874, #30346, #41694, .T. ) ;
#15329=ORIENTED_EDGE ( 'NONE', *, *, #12485, .T. ) ;
#15333=EDGE_LOOP ( 'NONE', ( #21053, #43023 ) ) ;
#15372=ORIENTED_EDGE ( 'NONE', *, *, #11420, .T. ) ;
#15378=CARTESIAN_POINT ( 'NONE',  ( 33.40854556226729954, -34.05525454449573175, -74.83297477053802993 ) ) ;
#15420=ORIENTED_EDGE ( 'NONE', *, *, #37480, .F. ) ;
#15454=CARTESIAN_POINT ( 'NONE',  ( -135.4416936590755540, -2.055254544495720648, -102.7350398871816424 ) ) ;
#15517=EDGE_LOOP ( 'NONE', ( #21894, #7242 ) ) ;
#15554=ORIENTED_EDGE ( 'NONE', *, *, #36160, .F. ) ;
#15557=DIRECTION ( 'NONE',  ( 1.000000000000000000, -3.035766082959410566E-17, 0.000000000000000000 ) ) ;
#15601=AXIS2_PLACEMENT_3D ( 'NONE', #1336, #5482, #4836 ) ;
#15686=LINE ( 'NONE', #22901, #33034 ) ;
#15703=CARTESIAN_POINT ( 'NONE',  ( 22.90854556226710415, -40.05525454449572464, -74.83297477053821467 ) ) ;
#15714=AXIS2_PLACEMENT_3D ( 'NONE', #7963, #40898, #17830 ) ;
#15729=ORIENTED_EDGE ( 'NONE', *, *, #10619, .F. ) ;
#15739=ADVANCED_FACE ( 'NONE', ( #27791 ), #37782, .T. ) ;
#15758=ORIENTED_EDGE ( 'NONE', *, *, #34930, .T. ) ;
#15762=DIRECTION ( 'NONE',  ( -1.000000000000000000, 3.942553354492743901E-17, 0.000000000000000000 ) ) ;
#15802=CARTESIAN_POINT ( 'NONE',  ( 56.25020680251638083, -2.055254544495725977, 2.972870684497274762 ) ) ;
#15816=VERTEX_POINT ( 'NONE', #31477 ) ;
#15846=AXIS2_PLACEMENT_3D ( 'NONE', #27835, #38050, #8380 ) ;
#15852=EDGE_CURVE ( 'NONE', #38270, #41456, #1193, .T. ) ;
#15860=DIRECTION ( 'NONE',  ( -3.009274222672345096E-17, -1.000000000000000000, 2.455023325076454960E-18 ) ) ;
#15875=AXIS2_PLACEMENT_3D ( 'NONE', #16420, #5180, #6357 ) ;
#15911=DIRECTION ( 'NONE',  ( 1.058513553088275437E-16, 1.000000000000000000, -8.813324511995299047E-17 ) ) ;
#15944=ADVANCED_FACE ( 'NONE', ( #29928 ), #33172, .T. ) ;
#15958=CARTESIAN_POINT ( 'NONE',  ( 31.80287614962791665, -40.05525454449572464, 69.29271901957253021 ) ) ;
#15975=CARTESIAN_POINT ( 'NONE',  ( -91.96080130434580724, -40.05525454449572464, 14.45886780445738218 ) ) ;
#15994=ORIENTED_EDGE ( 'NONE', *, *, #28713, .F. ) ;
#16052=CARTESIAN_POINT ( 'NONE',  ( 155.7547826636224499, -2.055254544495727309, 15.74958860255448734 ) ) ;
#16059=ORIENTED_EDGE ( 'NONE', *, *, #27178, .T. ) ;
#16075=CIRCLE ( 'NONE', #25828, 1.399999999999998579 ) ;
#16127=EDGE_LOOP ( 'NONE', ( #17251, #906, #13288, #12693 ) ) ;
#16136=CARTESIAN_POINT ( 'NONE',  ( 146.1418929693599580, -2.055254544495727309, -53.89157828313137344 ) ) ;
#16139=ORIENTED_EDGE ( 'NONE', *, *, #38151, .T. ) ;
#16141=FACE_BOUND ( 'NONE', #42568, .T. ) ;
#16146=DIRECTION ( 'NONE',  ( 1.000000000000000000, -3.009274222672345096E-17, 0.000000000000000000 ) ) ;
#16160=DIRECTION ( 'NONE',  ( -3.009274222672345096E-17, -1.000000000000000000, 2.455023325076454960E-18 ) ) ;
#16162=CIRCLE ( 'NONE', #1493, 16.00000000000023448 ) ;
#16199=DIRECTION ( 'NONE',  ( -1.058513553088275437E-16, -1.000000000000000000, 8.813324511995299047E-17 ) ) ;
#16212=CARTESIAN_POINT ( 'NONE',  ( -91.96080130434583566, -2.055254544495720648, 14.45886780445738395 ) ) ;
#16238=DIRECTION ( 'NONE',  ( 1.000000000000000000, -1.058513553088275437E-16, 0.000000000000000000 ) ) ;
#16252=DIRECTION ( 'NONE',  ( -1.000000000000000000, 0.000000000000000000, 0.000000000000000000 ) ) ;
#16272=ORIENTED_EDGE ( 'NONE', *, *, #27875, .F. ) ;
#16286=DIRECTION ( 'NONE',  ( -1.000000000000000000, 3.942553354492743901E-17, 0.000000000000000000 ) ) ;
#16295=DIRECTION ( 'NONE',  ( 1.000000000000000000, 0.000000000000000000, 0.000000000000000000 ) ) ;
#16322=FACE_OUTER_BOUND ( 'NONE', #42441, .T. ) ;
#16333=CIRCLE ( 'NONE', #972, 1.399999999999998579 ) ;
#16334=CARTESIAN_POINT ( 'NONE',  ( 42.80287614962790599, -40.05525454449572464, 69.29271901957253021 ) ) ;
#16336=CYLINDRICAL_SURFACE ( 'NONE', #41376, 11.00000000000023448 ) ;
#16373=CARTESIAN_POINT ( 'NONE',  ( 67.80287614962797704, -2.055254544495724645, 69.29271901957280022 ) ) ;
#16385=PLANE ( 'NONE',  #31621 ) ;
#16392=AXIS2_PLACEMENT_3D ( 'NONE', #32682, #2762, #42692 ) ;
#16397=LINE ( 'NONE', #188, #42390 ) ;
#16411=VERTEX_POINT ( 'NONE', #17642 ) ;
#16413=ADVANCED_FACE ( 'NONE', ( #10624 ), #7987, .T. ) ;
#16420=CARTESIAN_POINT ( 'NONE',  ( -79.93711883401132923, -12.05525454449572109, -145.8806300090334673 ) ) ;
#16453=DIRECTION ( 'NONE',  ( -3.009274222672345096E-17, -1.000000000000000000, 2.455023325076454960E-18 ) ) ;
#16457=AXIS2_PLACEMENT_3D ( 'NONE', #28555, #41608, #38328 ) ;
#16478=DIRECTION ( 'NONE',  ( -1.000000000000000000, 0.000000000000000000, 0.000000000000000000 ) ) ;
#16479=CARTESIAN_POINT ( 'NONE',  ( -102.4608013043457362, -35.35525454449571470, 14.45886780445633946 ) ) ;
#16481=ORIENTED_EDGE ( 'NONE', *, *, #30150, .T. ) ;
#16569=CARTESIAN_POINT ( 'NONE',  ( 33.40854556226729954, -35.35525454449573601, -74.83297477053802993 ) ) ;
#16575=ORIENTED_EDGE ( 'NONE', *, *, #24304, .F. ) ;
#16590=CARTESIAN_POINT ( 'NONE',  ( -97.01392236320388918, -12.05525454449572109, 76.75426063221412676 ) ) ;
#16593=CARTESIAN_POINT ( 'NONE',  ( 33.90854556226734218, -34.05525454449573175, -74.83297477053821467 ) ) ;
#16615=VECTOR ( 'NONE', #37902, 1000.000000000000000 ) ;
#16624=DIRECTION ( 'NONE',  ( -3.009274222672345096E-17, -1.000000000000000000, 2.455023325076455345E-18 ) ) ;
#16629=EDGE_LOOP ( 'NONE', ( #37865, #30082, #20609, #18365 ) ) ;
#16638=CIRCLE ( 'NONE', #33942, 10.99999999999998934 ) ;
#16694=ORIENTED_EDGE ( 'NONE', *, *, #8320, .T. ) ;
#16716=CARTESIAN_POINT ( 'NONE',  ( 42.80287614962790599, -12.05525454449572464, 69.29271901957253021 ) ) ;
#16777=DIRECTION ( 'NONE',  ( 3.009274222672345096E-17, 1.000000000000000000, -2.455023325076455345E-18 ) ) ;
#16843=DIRECTION ( 'NONE',  ( -3.009274222672345096E-17, -1.000000000000000000, 2.455023325076454960E-18 ) ) ;
#16849=LINE ( 'NONE', #11144, #34266 ) ;
#16856=ORIENTED_EDGE ( 'NONE', *, *, #4082, .F. ) ;
#16863=FACE_OUTER_BOUND ( 'NONE', #34501, .T. ) ;
#16869=DIRECTION ( 'NONE',  ( -1.000000000000000000, 3.469446951953615421E-17, 0.000000000000000000 ) ) ;
#16877=EDGE_LOOP ( 'NONE', ( #34000, #4655, #2450, #16928 ) ) ;
#16928=ORIENTED_EDGE ( 'NONE', *, *, #6160, .T. ) ;
#16955=DIRECTION ( 'NONE',  ( 2.731800627175558911E-17, 1.000000000000000000, -3.170996607629411740E-18 ) ) ;
#16957=EDGE_CURVE ( 'NONE', #39148, #2987, #20476, .T. ) ;
#16963=AXIS2_PLACEMENT_3D ( 'NONE', #30748, #13752, #10665 ) ;
#17011=ORIENTED_EDGE ( 'NONE', *, *, #25911, .F. ) ;
#17017=DIRECTION ( 'NONE',  ( 1.000000000000000000, -3.336006684570784581E-17, 0.000000000000000000 ) ) ;
#17048=EDGE_CURVE ( 'NONE', #1360, #2586, #24838, .T. ) ;
#17056=DIRECTION ( 'NONE',  ( -1.000000000000000000, 3.336006684570782732E-17, 0.000000000000000000 ) ) ;
#17068=CIRCLE ( 'NONE', #19162, 99.99999999999994316 ) ;
#17088=LINE ( 'NONE', #30378, #41463 ) ;
#17138=ORIENTED_EDGE ( 'NONE', *, *, #4082, .T. ) ;
#17163=CIRCLE ( 'NONE', #479, 10.49999999999999467 ) ;
#17226=AXIS2_PLACEMENT_3D ( 'NONE', #35463, #5371, #32198 ) ;
#17227=EDGE_CURVE ( 'NONE', #41341, #23828, #6712, .T. ) ;
#17238=( NAMED_UNIT ( * ) PLANE_ANGLE_UNIT ( ) SI_UNIT ( $, .RADIAN. ) );
#17251=ORIENTED_EDGE ( 'NONE', *, *, #27755, .F. ) ;
#17258=EDGE_CURVE ( 'NONE', #1626, #38421, #26942, .T. ) ;
#17261=AXIS2_PLACEMENT_3D ( 'NONE', #22973, #12694, #19905 ) ;
#17272=LINE ( 'NONE', #37507, #29723 ) ;
#17274=ORIENTED_EDGE ( 'NONE', *, *, #27875, .T. ) ;
#17328=ORIENTED_EDGE ( 'NONE', *, *, #14218, .T. ) ;
#17342=DIRECTION ( 'NONE',  ( 1.000000000000000000, -3.469446951953614189E-17, 0.000000000000000000 ) ) ;
#17378=( LENGTH_UNIT ( ) NAMED_UNIT ( * ) SI_UNIT ( .MILLI., .METRE. ) );
#17398=CARTESIAN_POINT ( 'NONE',  ( 42.80287614962790599, -40.05525454449572464, 69.29271901957253021 ) ) ;
#17412=ORIENTED_EDGE ( 'NONE', *, *, #25107, .T. ) ;
#17456=DIRECTION ( 'NONE',  ( -1.000000000000000000, 1.084202172485488534E-16, 0.000000000000000000 ) ) ;
#17457=FACE_OUTER_BOUND ( 'NONE', #11578, .T. ) ;
#17494=VERTEX_POINT ( 'NONE', #938 ) ;
#17502=ORIENTED_EDGE ( 'NONE', *, *, #9336, .F. ) ;
#17515=AXIS2_PLACEMENT_3D ( 'NONE', #11715, #25048, #8407 ) ;
#17546=VERTEX_POINT ( 'NONE', #8165 ) ;
#17558=DIRECTION ( 'NONE',  ( 3.009274222672345096E-17, 1.000000000000000000, -2.455023325076455345E-18 ) ) ;
#17562=ORIENTED_EDGE ( 'NONE', *, *, #25107, .F. ) ;
#17564=CIRCLE ( 'NONE', #27276, 11.00000000000023803 ) ;
#17580=EDGE_CURVE ( 'NONE', #23370, #34600, #22831, .T. ) ;
#17591=FILL_AREA_STYLE_COLOUR ( '', #40776 ) ;
#17642=CARTESIAN_POINT ( 'NONE',  ( 52.26814377733353467, -2.055254544495723756, -19.42827587850796434 ) ) ;
#17655=VERTEX_POINT ( 'NONE', #17804 ) ;
#17694=FACE_BOUND ( 'NONE', #31234, .T. ) ;
#17699=ORIENTED_EDGE ( 'NONE', *, *, #32084, .F. ) ;
#17705=ORIENTED_EDGE ( 'NONE', *, *, #34165, .T. ) ;
#17716=EDGE_CURVE ( 'NONE', #28510, #37542, #12308, .T. ) ;
#17747=PRODUCT_DEFINITION_FORMATION_WITH_SPECIFIED_SOURCE ( 'ANY', '', #33245, .NOT_KNOWN. ) ;
#17758=ORIENTED_EDGE ( 'NONE', *, *, #34930, .F. ) ;
#17760=DIRECTION ( 'NONE',  ( 1.000000000000000000, 0.000000000000000000, 0.000000000000000000 ) ) ;
#17804=CARTESIAN_POINT ( 'NONE',  ( -100.6569797752917879, -2.055254544495720648, -8.979913733870429127 ) ) ;
#17812=DIRECTION ( 'NONE',  ( -3.009274222672345712E-17, -1.000000000000000000, 2.455023325076455345E-18 ) ) ;
#17830=DIRECTION ( 'NONE',  ( 1.000000000000000000, 0.000000000000000000, 0.000000000000000000 ) ) ;
#17893=CARTESIAN_POINT ( 'NONE',  ( 22.90854556226710415, -14.05525454449572997, -74.83297477053821467 ) ) ;
#17946=ORIENTED_EDGE ( 'NONE', *, *, #8889, .F. ) ;
#17951=CARTESIAN_POINT ( 'NONE',  ( 22.90854556226710415, -12.05525454449572464, -74.83297477053821467 ) ) ;
#18042=DIRECTION ( 'NONE',  ( -1.058513553088275437E-16, -1.000000000000000000, 8.813324511995299047E-17 ) ) ;
#18060=ORIENTED_EDGE ( 'NONE', *, *, #31338, .T. ) ;
#18113=AXIS2_PLACEMENT_3D ( 'NONE', #18202, #14040, #27998 ) ;
#18115=CARTESIAN_POINT ( 'NONE',  ( 12.40854556226731198, -35.35525454449573601, -74.83297477053802993 ) ) ;
#18139=CIRCLE ( 'NONE', #20209, 10.99999999999999645 ) ;
#18202=CARTESIAN_POINT ( 'NONE',  ( -8.749793197483592522, 117.9447454555042754, 2.972870684497274762 ) ) ;
#18221=CYLINDRICAL_SURFACE ( 'NONE', #19663, 10.99999999999999645 ) ;
#18260=CARTESIAN_POINT ( 'NONE',  ( -26.14979319748359643, -2.055254544495722868, 2.972870684497277427 ) ) ;
#18261=ORIENTED_EDGE ( 'NONE', *, *, #36153, .F. ) ;
#18262=ORIENTED_EDGE ( 'NONE', *, *, #42066, .T. ) ;
#18270=FACE_OUTER_BOUND ( 'NONE', #11926, .T. ) ;
#18362=VERTEX_POINT ( 'NONE', #40111 ) ;
#18365=ORIENTED_EDGE ( 'NONE', *, *, #25735, .T. ) ;
#18373=DIRECTION ( 'NONE',  ( 3.009274222672345096E-17, 1.000000000000000000, -2.455023325076454960E-18 ) ) ;
#18429=CARTESIAN_POINT ( 'NONE',  ( -8.749793197483594298, -2.055254544495723756, 2.972870684497274762 ) ) ;
#18430=ORIENTED_EDGE ( 'NONE', *, *, #22811, .T. ) ;
#18451=ORIENTED_EDGE ( 'NONE', *, *, #36206, .T. ) ;
#18453=ORIENTED_EDGE ( 'NONE', *, *, #87, .F. ) ;
#18480=CYLINDRICAL_SURFACE ( 'NONE', #2116, 100.0000000000000000 ) ;
#18500=EDGE_CURVE ( 'NONE', #24559, #39731, #34232, .T. ) ;
#18513=ORIENTED_EDGE ( 'NONE', *, *, #43083, .F. ) ;
#18529=VERTEX_POINT ( 'NONE', #37074 ) ;
#18533=CARTESIAN_POINT ( 'NONE',  ( -8.749793197483594298, -12.05525454449572464, 2.972870684497274762 ) ) ;
#18572=CYLINDRICAL_SURFACE ( 'NONE', #7666, 10.49999999999999467 ) ;
#18619=DIRECTION ( 'NONE',  ( -1.000000000000000000, 1.577021341797097807E-16, 0.000000000000000000 ) ) ;
#18648=CIRCLE ( 'NONE', #39492, 1.399999999999998579 ) ;
#18654=ADVANCED_FACE ( 'NONE', ( #24459 ), #24671, .T. ) ;
#18668=CARTESIAN_POINT ( 'NONE',  ( -91.96080130434580724, -14.05525454449571043, 14.45886780445738218 ) ) ;
#18686=CARTESIAN_POINT ( 'NONE',  ( 53.30287614962722387, -35.35525454449572180, 69.29271901957299917 ) ) ;
#18700=DIRECTION ( 'NONE',  ( 1.000000000000000000, -1.058513553088275437E-16, 0.000000000000000000 ) ) ;
#18761=DIRECTION ( 'NONE',  ( -1.000000000000000000, 2.668805347656627603E-17, 0.000000000000000000 ) ) ;
#18797=DIRECTION ( 'NONE',  ( 2.932542530036133930E-17, 1.000000000000000000, -5.216001792149171863E-18 ) ) ;
#18808=VERTEX_POINT ( 'NONE', #18998 ) ;
#18867=CARTESIAN_POINT ( 'NONE',  ( 2.250206802516403481, -2.055254544495723312, 2.972870684497274762 ) ) ;
#18902=CARTESIAN_POINT ( 'NONE',  ( 22.90854556226730310, -34.05525454449573175, -74.83297477053802993 ) ) ;
#18912=AXIS2_PLACEMENT_3D ( 'NONE', #7149, #3646, #9580 ) ;
#18914=FACE_OUTER_BOUND ( 'NONE', #41590, .T. ) ;
#18957=DIRECTION ( 'NONE',  ( 1.000000000000000000, 0.000000000000000000, 0.000000000000000000 ) ) ;
#18968=VECTOR ( 'NONE', #19697, 1000.000000000000000 ) ;
#18998=CARTESIAN_POINT ( 'NONE',  ( 47.90854556226721428, -12.05525454449572464, -74.83297477053847047 ) ) ;
#19013=DIRECTION ( 'NONE',  ( 1.000000000000000000, -3.336006684570782732E-17, 0.000000000000000000 ) ) ;
#19043=ORIENTED_EDGE ( 'NONE', *, *, #20371, .F. ) ;
#19050=AXIS2_PLACEMENT_3D ( 'NONE', #21599, #4510, #38326 ) ;
#19076=VERTEX_POINT ( 'NONE', #7942 ) ;
#19116=ORIENTED_EDGE ( 'NONE', *, *, #24304, .T. ) ;
#19129=DIRECTION ( 'NONE',  ( -1.000000000000000000, 3.469446951953614189E-17, 0.000000000000000000 ) ) ;
#19162=AXIS2_PLACEMENT_3D ( 'NONE', #36144, #6465, #19188 ) ;
#19188=DIRECTION ( 'NONE',  ( 1.000000000000000000, -3.035766082959414264E-17, 0.000000000000000000 ) ) ;
#19198=VERTEX_POINT ( 'NONE', #5949 ) ;
#19202=FACE_OUTER_BOUND ( 'NONE', #38329, .T. ) ;
#19204=DIRECTION ( 'NONE',  ( -1.000000000000000000, 0.000000000000000000, 0.000000000000000000 ) ) ;
#19212=CIRCLE ( 'NONE', #329, 16.00000000000023448 ) ;
#19221=DIRECTION ( 'NONE',  ( -3.009274222672345096E-17, -1.000000000000000000, 2.455023325076454960E-18 ) ) ;
#19275=DIRECTION ( 'NONE',  ( -3.009274222672345096E-17, -1.000000000000000000, 2.455023325076454960E-18 ) ) ;
#19290=VERTEX_POINT ( 'NONE', #9234 ) ;
#19325=EDGE_LOOP ( 'NONE', ( #36930, #15329 ) ) ;
#19395=VERTEX_POINT ( 'NONE', #40174 ) ;
#19409=ORIENTED_EDGE ( 'NONE', *, *, #21561, .F. ) ;
#19413=ORIENTED_EDGE ( 'NONE', *, *, #11420, .F. ) ;
#19421=DIRECTION ( 'NONE',  ( -1.000000000000000000, 0.000000000000000000, 0.000000000000000000 ) ) ;
#19434=ORIENTED_EDGE ( 'NONE', *, *, #29652, .T. ) ;
#19455=CIRCLE ( 'NONE', #11791, 65.00000000000000000 ) ;
#19470=DIRECTION ( 'NONE',  ( 1.000000000000000000, 0.000000000000000000, 0.000000000000000000 ) ) ;
#19544=CARTESIAN_POINT ( 'NONE',  ( -102.9608013043458072, -40.05525454449572464, 14.45886780445738218 ) ) ;
#19547=FACE_OUTER_BOUND ( 'NONE', #40610, .T. ) ;
#19567=DIRECTION ( 'NONE',  ( -1.000000000000000000, 1.577021341797098793E-16, 0.000000000000000000 ) ) ;
#19578=EDGE_CURVE ( 'NONE', #30346, #9874, #36166, .T. ) ;
#19622=FACE_OUTER_BOUND ( 'NONE', #7416, .T. ) ;
#19631=LINE ( 'NONE', #6714, #33348 ) ;
#19633=AXIS2_PLACEMENT_3D ( 'NONE', #41380, #8663, #31166 ) ;
#19639=EDGE_CURVE ( 'NONE', #9213, #4169, #9708, .T. ) ;
#19640=VERTEX_POINT ( 'NONE', #8974 ) ;
#19643=ORIENTED_EDGE ( 'NONE', *, *, #35137, .T. ) ;
#19649=ORIENTED_EDGE ( 'NONE', *, *, #31170, .F. ) ;
#19663=AXIS2_PLACEMENT_3D ( 'NONE', #1576, #11423, #28229 ) ;
#19675=ORIENTED_EDGE ( 'NONE', *, *, #3600, .T. ) ;
#19697=DIRECTION ( 'NONE',  ( -3.009274222672345096E-17, -1.000000000000000000, 2.455023325076454960E-18 ) ) ;
#19791=VECTOR ( 'NONE', #31768, 1000.000000000000000 ) ;
#19828=ORIENTED_EDGE ( 'NONE', *, *, #27314, .F. ) ;
#19866=FACE_OUTER_BOUND ( 'NONE', #35811, .T. ) ;
#19871=ORIENTED_EDGE ( 'NONE', *, *, #14324, .T. ) ;
#19901=DIRECTION ( 'NONE',  ( -3.009274222672345096E-17, -1.000000000000000000, 2.455023325076454960E-18 ) ) ;
#19905=DIRECTION ( 'NONE',  ( 1.000000000000000000, -3.009274222672345096E-17, 0.000000000000000000 ) ) ;
#19908=ORIENTED_EDGE ( 'NONE', *, *, #3600, .F. ) ;
#19914=FACE_BOUND ( 'NONE', #28544, .T. ) ;
#19919=DIRECTION ( 'NONE',  ( 1.000000000000000000, 0.000000000000000000, 0.000000000000000000 ) ) ;
#19987=DIRECTION ( 'NONE',  ( 3.009274222672345096E-17, 1.000000000000000000, -2.455023325076454960E-18 ) ) ;
#19996=AXIS2_PLACEMENT_3D ( 'NONE', #39355, #9063, #2275 ) ;
#20026=AXIS2_PLACEMENT_3D ( 'NONE', #23070, #29379, #22226 ) ;
#20066=AXIS2_PLACEMENT_3D ( 'NONE', #36269, #42398, #9881 ) ;
#20078=DIRECTION ( 'NONE',  ( -3.009274222672345096E-17, -1.000000000000000000, 2.455023325076455345E-18 ) ) ;
#20084=ORIENTED_EDGE ( 'NONE', *, *, #29566, .F. ) ;
#20104=CARTESIAN_POINT ( 'NONE',  ( 11.90854556226686789, -40.05525454449572464, -74.83297477053821467 ) ) ;
#20141=DIRECTION ( 'NONE',  ( 1.000000000000000000, 0.000000000000000000, 0.000000000000000000 ) ) ;
#20143=DIRECTION ( 'NONE',  ( -1.058513553088275437E-16, -1.000000000000000000, 8.813324511995299047E-17 ) ) ;
#20145=CYLINDRICAL_SURFACE ( 'NONE', #20378, 24.99999999999999289 ) ;
#20146=FACE_OUTER_BOUND ( 'NONE', #26284, .T. ) ;
#20203=ORIENTED_EDGE ( 'NONE', *, *, #21847, .F. ) ;
#20209=AXIS2_PLACEMENT_3D ( 'NONE', #13888, #37188, #10811 ) ;
#20263=AXIS2_PLACEMENT_3D ( 'NONE', #25039, #34800, #8188 ) ;
#20371=EDGE_CURVE ( 'NONE', #19640, #33033, #19631, .T. ) ;
#20378=AXIS2_PLACEMENT_3D ( 'NONE', #33404, #3487, #21870 ) ;
#20380=VECTOR ( 'NONE', #7457, 1000.000000000000000 ) ;
#20382=CYLINDRICAL_SURFACE ( 'NONE', #3286, 64.99999999999998579 ) ;
#20426=SURFACE_SIDE_STYLE ('',( #726 ) ) ;
#20428=CARTESIAN_POINT ( 'NONE',  ( -58.65872368235312706, -12.05525454449572109, -38.66963954070958209 ) ) ;
#20461=ORIENTED_EDGE ( 'NONE', *, *, #2146, .T. ) ;
#20476=LINE ( 'NONE', #27428, #27603 ) ;
#20562=ORIENTED_EDGE ( 'NONE', *, *, #29362, .T. ) ;
#20580=CIRCLE ( 'NONE', #31017, 64.99999999999997158 ) ;
#20609=ORIENTED_EDGE ( 'NONE', *, *, #28713, .T. ) ;
#20624=AXIS2_PLACEMENT_3D ( 'NONE', #33266, #40639, #36738 ) ;
#20630=AXIS2_PLACEMENT_3D ( 'NONE', #36264, #13396, #16238 ) ;
#20654=AXIS2_PLACEMENT_3D ( 'NONE', #27827, #37818, #5094 ) ;
#20668=FACE_OUTER_BOUND ( 'NONE', #12094, .T. ) ;
#20710=LINE ( 'NONE', #33754, #23503 ) ;
#20727=SURFACE_STYLE_FILL_AREA ( #1019 ) ;
#20882=EDGE_CURVE ( 'NONE', #33446, #2987, #18139, .T. ) ;
#20916=DIRECTION ( 'NONE',  ( -3.009274222672345096E-17, -1.000000000000000000, 2.455023325076454960E-18 ) ) ;
#20958=CIRCLE ( 'NONE', #35533, 10.99999999999999645 ) ;
#20963=ORIENTED_EDGE ( 'NONE', *, *, #37999, .F. ) ;
#20971=EDGE_LOOP ( 'NONE', ( #32783, #26974, #40612, #15758 ) ) ;
#21053=ORIENTED_EDGE ( 'NONE', *, *, #20882, .T. ) ;
#21066=ORIENTED_EDGE ( 'NONE', *, *, #22811, .F. ) ;
#21088=CIRCLE ( 'NONE', #2872, 10.99999999999998934 ) ;
#21092=ORIENTED_EDGE ( 'NONE', *, *, #27184, .F. ) ;
#21147=ORIENTED_EDGE ( 'NONE', *, *, #6683, .T. ) ;
#21175=EDGE_CURVE ( 'NONE', #27084, #18808, #17088, .T. ) ;
#21225=ADVANCED_FACE ( 'NONE', ( #16322, #1543 ), #38992, .F. ) ;
#21242=( GEOMETRIC_REPRESENTATION_CONTEXT ( 3 ) GLOBAL_UNCERTAINTY_ASSIGNED_CONTEXT ( ( #10384 ) ) GLOBAL_UNIT_ASSIGNED_CONTEXT ( ( #23770, #27241, #4512 ) ) REPRESENTATION_CONTEXT ( 'NONE', 'WORKASPACE' ) );
#21250=CIRCLE ( 'NONE', #2362, 100.0000000000000000 ) ;
#21268=FACE_OUTER_BOUND ( 'NONE', #24428, .T. ) ;
#21273=ORIENTED_EDGE ( 'NONE', *, *, #19578, .T. ) ;
#21312=LINE ( 'NONE', #34561, #30473 ) ;
#21399=VECTOR ( 'NONE', #1452, 1000.000000000000000 ) ;
#21419=CARTESIAN_POINT ( 'NONE',  ( -91.96080130434583566, -2.055254544495720648, 14.45886780445738395 ) ) ;
#21439=CARTESIAN_POINT ( 'NONE',  ( 33.90854556226734218, -40.05525454449572464, -74.83297477053821467 ) ) ;
#21470=DIRECTION ( 'NONE',  ( 3.009274222672345096E-17, 1.000000000000000000, -2.455023325076454960E-18 ) ) ;
#21483=CIRCLE ( 'NONE', #29101, 10.99999999999998934 ) ;
#21525=EDGE_LOOP ( 'NONE', ( #8676, #38458 ) ) ;
#21559=ADVANCED_FACE ( 'NONE', ( #35363 ), #4608, .T. ) ;
#21561=EDGE_CURVE ( 'NONE', #30653, #42446, #37177, .T. ) ;
#21566=DIRECTION ( 'NONE',  ( 3.009274222672345096E-17, 1.000000000000000000, -2.455023325076454960E-18 ) ) ;
#21599=CARTESIAN_POINT ( 'NONE',  ( -8.749793197483592522, 117.9447454555042754, 2.972870684497274762 ) ) ;
#21653=DIRECTION ( 'NONE',  ( -1.000000000000000000, 3.469446951953611724E-17, 0.000000000000000000 ) ) ;
#21662=DIRECTION ( 'NONE',  ( -3.009274222672345096E-17, -1.000000000000000000, 2.455023325076454960E-18 ) ) ;
#21671=DIRECTION ( 'NONE',  ( -3.009274222672345096E-17, -1.000000000000000000, 2.455023325076454960E-18 ) ) ;
#21699=CIRCLE ( 'NONE', #40433, 25.00000000000000000 ) ;
#21719=ADVANCED_FACE ( 'NONE', ( #12892, #22315 ), #16385, .F. ) ;
#21731=VERTEX_POINT ( 'NONE', #13769 ) ;
#21746=EDGE_CURVE ( 'NONE', #34600, #22843, #36861, .T. ) ;
#21763=UNCERTAINTY_MEASURE_WITH_UNIT (LENGTH_MEASURE( 1.000000000000000082E-05 ), #33766, 'distance_accuracy_value', 'NONE');
#21816=CARTESIAN_POINT ( 'NONE',  ( 42.80287614962790599, -12.05525454449571932, 69.29271901957253021 ) ) ;
#21847=EDGE_CURVE ( 'NONE', #14319, #32706, #10918, .T. ) ;
#21861=VECTOR ( 'NONE', #27412, 1000.000000000000000 ) ;
#21869=ORIENTED_EDGE ( 'NONE', *, *, #42066, .F. ) ;
#21870=DIRECTION ( 'NONE',  ( 1.000000000000000000, -3.469446951953615421E-17, 0.000000000000000000 ) ) ;
#21894=ORIENTED_EDGE ( 'NONE', *, *, #29295, .F. ) ;
#21900=DIRECTION ( 'NONE',  ( 1.000000000000000000, -3.035766082959412415E-17, 0.000000000000000000 ) ) ;
#21926=CIRCLE ( 'NONE', #27466, 10.99999999999999645 ) ;
#21939=AXIS2_PLACEMENT_3D ( 'NONE', #38143, #11992, #5193 ) ;
#21944=ORIENTED_EDGE ( 'NONE', *, *, #13896, .T. ) ;
#21956=AXIS2_PLACEMENT_3D ( 'NONE', #34484, #21671, #5037 ) ;
#21968=AXIS2_PLACEMENT_3D ( 'NONE', #1055, #37509, #36463 ) ;
#22028=AXIS2_PLACEMENT_3D ( 'NONE', #26140, #15911, #5627 ) ;
#22073=DIRECTION ( 'NONE',  ( -3.009274222672345096E-17, -1.000000000000000000, 2.455023325076454960E-18 ) ) ;
#22107=ADVANCED_FACE ( 'NONE', ( #12634 ), #16336, .T. ) ;
#22108=ORIENTED_EDGE ( 'NONE', *, *, #8656, .T. ) ;
#22118=CARTESIAN_POINT ( 'NONE',  ( -8.749793197483596074, -2.055254544495723312, 2.972870684497275207 ) ) ;
#22133=FACE_BOUND ( 'NONE', #38881, .T. ) ;
#22178=DIRECTION ( 'NONE',  ( -3.009274222672345096E-17, -1.000000000000000000, 2.455023325076454960E-18 ) ) ;
#22226=DIRECTION ( 'NONE',  ( 1.000000000000000000, 0.000000000000000000, 0.000000000000000000 ) ) ;
#22229=EDGE_LOOP ( 'NONE', ( #12442, #4257 ) ) ;
#22235=CARTESIAN_POINT ( 'NONE',  ( -8.749793197483592522, 117.9447454555042754, 2.972870684497274762 ) ) ;
#22315=FACE_BOUND ( 'NONE', #3055, .T. ) ;
#22387=CYLINDRICAL_SURFACE ( 'NONE', #27163, 64.99999999999997158 ) ;
#22388=ORIENTED_EDGE ( 'NONE', *, *, #8656, .F. ) ;
#22408=CARTESIAN_POINT ( 'NONE',  ( 11.90854556226686789, -40.05525454449572464, -74.83297477053821467 ) ) ;
#22410=ORIENTED_EDGE ( 'NONE', *, *, #2898, .T. ) ;
#22494=CARTESIAN_POINT ( 'NONE',  ( -8.749793197483594298, -12.05525454449572464, 2.972870684497274762 ) ) ;
#22518=LINE ( 'NONE', #15958, #5255 ) ;
#22529=EDGE_LOOP ( 'NONE', ( #16272, #12706 ) ) ;
#22541=VECTOR ( 'NONE', #33364, 1000.000000000000000 ) ;
#22639=ORIENTED_EDGE ( 'NONE', *, *, #37999, .T. ) ;
#22645=AXIS2_PLACEMENT_3D ( 'NONE', #4546, #7834, #29744 ) ;
#22673=DIRECTION ( 'NONE',  ( -3.009274222672345096E-17, -1.000000000000000000, 2.455023325076454960E-18 ) ) ;
#22687=PLANE ( 'NONE',  #16392 ) ;
#22706=FACE_OUTER_BOUND ( 'NONE', #33370, .T. ) ;
#22719=CARTESIAN_POINT ( 'NONE',  ( 65.39325745242679488, -12.05525454449572464, 58.58409293616905700 ) ) ;
#22722=PRODUCT_CONTEXT ( 'NONE', #26721, 'mechanical' ) ;
#22725=DIRECTION ( 'NONE',  ( 1.000000000000000000, 0.000000000000000000, 0.000000000000000000 ) ) ;
#22726=ORIENTED_EDGE ( 'NONE', *, *, #37157, .F. ) ;
#22728=AXIS2_PLACEMENT_3D ( 'NONE', #42094, #12246, #25575 ) ;
#22811=EDGE_CURVE ( 'NONE', #41456, #38270, #8690, .T. ) ;
#22831=CIRCLE ( 'NONE', #14438, 1.399999999999998579 ) ;
#22843=VERTEX_POINT ( 'NONE', #18260 ) ;
#22845=CIRCLE ( 'NONE', #3966, 100.0000000000000000 ) ;
#22901=CARTESIAN_POINT ( 'NONE',  ( 47.55521504368574881, -2.055254544495723756, -70.64469547305695585 ) ) ;
#22913=LINE ( 'NONE', #16569, #13010 ) ;
#22973=CARTESIAN_POINT ( 'NONE',  ( 42.80287614962790599, -40.05525454449572464, 69.29271901957253021 ) ) ;
#23026=DIRECTION ( 'NONE',  ( 1.000000000000000000, -3.336006684570784581E-17, 0.000000000000000000 ) ) ;
#23037=ADVANCED_FACE ( 'NONE', ( #32159, #32584 ), #2040, .T. ) ;
#23038=CIRCLE ( 'NONE', #33428, 64.99999999999998579 ) ;
#23070=CARTESIAN_POINT ( 'NONE',  ( 22.90854556226710415, -35.35525454449573601, -74.83297477053821467 ) ) ;
#23140=DIRECTION ( 'NONE',  ( -1.058513553088275437E-16, -1.000000000000000000, 8.813324511995299047E-17 ) ) ;
#23192=FACE_OUTER_BOUND ( 'NONE', #7644, .T. ) ;
#23201=VERTEX_POINT ( 'NONE', #29974 ) ;
#23225=DIRECTION ( 'NONE',  ( 1.058513553088275437E-16, 1.000000000000000000, -8.813324511995299047E-17 ) ) ;
#23267=ADVANCED_FACE ( 'NONE', ( #32998, #238 ), #3085, .T. ) ;
#23311=EDGE_LOOP ( 'NONE', ( #6891, #25633 ) ) ;
#23370=VERTEX_POINT ( 'NONE', #34738 ) ;
#23388=EDGE_CURVE ( 'NONE', #31096, #19076, #40815, .T. ) ;
#23400=CIRCLE ( 'NONE', #4543, 10.99999999999999645 ) ;
#23422=ORIENTED_EDGE ( 'NONE', *, *, #17580, .T. ) ;
#23433=ORIENTED_EDGE ( 'NONE', *, *, #27416, .T. ) ;
#23435=CARTESIAN_POINT ( 'NONE',  ( -8.749793197483594298, -2.055254544495723756, 2.972870684497274762 ) ) ;
#23503=VECTOR ( 'NONE', #134, 1000.000000000000000 ) ;
#23574=ORIENTED_EDGE ( 'NONE', *, *, #12746, .F. ) ;
#23592=ADVANCED_FACE ( 'NONE', ( #28213 ), #8543, .F. ) ;
#23603=ORIENTED_EDGE ( 'NONE', *, *, #5601, .F. ) ;
#23629=CIRCLE ( 'NONE', #33346, 100.0000000000000000 ) ;
#23651=CARTESIAN_POINT ( 'NONE',  ( 6.908545562266867002, -12.05525454449572997, -74.83297477053821467 ) ) ;
#23699=CARTESIAN_POINT ( 'NONE',  ( -91.96080130434580724, -14.05525454449571043, 14.45886780445738218 ) ) ;
#23732=CARTESIAN_POINT ( 'NONE',  ( -45.51113419504475388, -2.055254544495720648, 56.57887602028989704 ) ) ;
#23770=( LENGTH_UNIT ( ) NAMED_UNIT ( * ) SI_UNIT ( .MILLI., .METRE. ) );
#23785=DIRECTION ( 'NONE',  ( -1.000000000000000000, 0.000000000000000000, 0.000000000000000000 ) ) ;
#23810=EDGE_CURVE ( 'NONE', #10648, #34172, #5165, .T. ) ;
#23828=VERTEX_POINT ( 'NONE', #14592 ) ;
#23836=AXIS2_PLACEMENT_3D ( 'NONE', #21816, #11529, #1462 ) ;
#23915=DIRECTION ( 'NONE',  ( 3.009274222672345096E-17, 1.000000000000000000, -2.455023325076454960E-18 ) ) ;
#23917=EDGE_LOOP ( 'NONE', ( #14354, #11297, #24090, #35752 ) ) ;
#23926=CARTESIAN_POINT ( 'NONE',  ( 2.250206802516407034, 117.9447454555042754, 2.972870684497274762 ) ) ;
#24005=ORIENTED_EDGE ( 'NONE', *, *, #37983, .T. ) ;
#24047=ORIENTED_EDGE ( 'NONE', *, *, #736, .T. ) ;
#24090=ORIENTED_EDGE ( 'NONE', *, *, #24737, .T. ) ;
#24171=CARTESIAN_POINT ( 'NONE',  ( 58.80287614962789888, -14.05525454449572109, 69.29271901957253021 ) ) ;
#24200=ORIENTED_EDGE ( 'NONE', *, *, #6160, .F. ) ;
#24212=FILL_AREA_STYLE_COLOUR ( '', #31664 ) ;
#24240=CIRCLE ( 'NONE', #5394, 10.49999999999999467 ) ;
#24244=EDGE_CURVE ( 'NONE', #37542, #39731, #1867, .T. ) ;
#24283=CARTESIAN_POINT ( 'NONE',  ( -24.74979319748359785, 5.944745455504278020, 2.972870684497277427 ) ) ;
#24304=EDGE_CURVE ( 'NONE', #6283, #28510, #40873, .T. ) ;
#24305=ADVANCED_FACE ( 'NONE', ( #42506 ), #6088, .T. ) ;
#24378=UNCERTAINTY_MEASURE_WITH_UNIT (LENGTH_MEASURE( 1.000000000000000082E-05 ), #17378, 'distance_accuracy_value', 'NONE');
#24379=EDGE_LOOP ( 'NONE', ( #39548, #21944, #31431, #15994 ) ) ;
#24402=DIRECTION ( 'NONE',  ( 3.009274222672345096E-17, 1.000000000000000000, -2.455023325076455345E-18 ) ) ;
#24409=CARTESIAN_POINT ( 'NONE',  ( -80.96080130434580724, -40.05525454449572464, 14.45886780445738395 ) ) ;
#24428=EDGE_LOOP ( 'NONE', ( #19649, #26893, #18262, #26121 ) ) ;
#24459=FACE_OUTER_BOUND ( 'NONE', #2242, .T. ) ;
#24559=VERTEX_POINT ( 'NONE', #27545 ) ;
#24574=DIRECTION ( 'NONE',  ( -1.058513553088275437E-16, -1.000000000000000000, 8.813324511995299047E-17 ) ) ;
#24578=EDGE_CURVE ( 'NONE', #9874, #41456, #40818, .T. ) ;
#24580=DIRECTION ( 'NONE',  ( -3.009274222672345096E-17, -1.000000000000000000, 2.455023325076454960E-18 ) ) ;
#24586=DIRECTION ( 'NONE',  ( -1.000000000000000000, 0.000000000000000000, 0.000000000000000000 ) ) ;
#24613=VERTEX_POINT ( 'NONE', #39793 ) ;
#24626=DIRECTION ( 'NONE',  ( 1.058513553088275437E-16, 1.000000000000000000, -8.813324511995299047E-17 ) ) ;
#24627=ORIENTED_EDGE ( 'NONE', *, *, #24244, .T. ) ;
#24662=DIRECTION ( 'NONE',  ( -1.000000000000000000, 0.000000000000000000, 0.000000000000000000 ) ) ;
#24671=CYLINDRICAL_SURFACE ( 'NONE', #35400, 25.00000000000002132 ) ;
#24675=CARTESIAN_POINT ( 'NONE',  ( -91.96080130434573618, -35.35525454449571470, 14.45886780445633946 ) ) ;
#24731=ORIENTED_EDGE ( 'NONE', *, *, #9813, .F. ) ;
#24737=EDGE_CURVE ( 'NONE', #43113, #18362, #17163, .T. ) ;
#24742=EDGE_CURVE ( 'NONE', #40515, #17655, #22845, .T. ) ;
#24765=DIRECTION ( 'NONE',  ( -3.009274222672345096E-17, -1.000000000000000000, 2.455023325076454960E-18 ) ) ;
#24770=CIRCLE ( 'NONE', #6577, 10.49999999999999467 ) ;
#24838=LINE ( 'NONE', #38092, #36629 ) ;
#24877=CIRCLE ( 'NONE', #32479, 25.00000000000002132 ) ;
#24882=ORIENTED_EDGE ( 'NONE', *, *, #7080, .F. ) ;
#24892=CARTESIAN_POINT ( 'NONE',  ( 42.80287614962796994, -12.05525454449572464, 69.29271901957280022 ) ) ;
#24930=CARTESIAN_POINT ( 'NONE',  ( 22.90854556226710415, -40.05525454449572464, -74.83297477053821467 ) ) ;
#24935=AXIS2_PLACEMENT_3D ( 'NONE', #30979, #5388, #18957 ) ;
#24954=CARTESIAN_POINT ( 'NONE',  ( 42.80287614962723808, -35.35525454449572180, 69.29271901957299917 ) ) ;
#24977=ORIENTED_EDGE ( 'NONE', *, *, #12137, .F. ) ;
#24996=VECTOR ( 'NONE', #3890, 1000.000000000000000 ) ;
#25011=LINE ( 'NONE', #18686, #35280 ) ;
#25016=ADVANCED_FACE ( 'NONE', ( #20146 ), #7646, .T. ) ;
#25032=VECTOR ( 'NONE', #12715, 1000.000000000000000 ) ;
#25039=CARTESIAN_POINT ( 'NONE',  ( -91.96080130434573618, -34.05525454449571043, 14.45886780445633946 ) ) ;
#25048=DIRECTION ( 'NONE',  ( -1.058513553088275437E-16, -1.000000000000000000, 8.813324511995299047E-17 ) ) ;
#25075=CARTESIAN_POINT ( 'NONE',  ( 42.80287614962790599, -14.05525454449571932, 69.29271901957253021 ) ) ;
#25089=ORIENTED_EDGE ( 'NONE', *, *, #24737, .F. ) ;
#25107=EDGE_CURVE ( 'NONE', #39162, #41904, #15097, .T. ) ;
#25118=ADVANCED_FACE ( 'NONE', ( #41225 ), #5026, .T. ) ;
#25181=EDGE_LOOP ( 'NONE', ( #43096, #1984, #41050, #16139 ) ) ;
#25182=CARTESIAN_POINT ( 'NONE',  ( 22.90854556226710415, -40.05525454449572464, -74.83297477053821467 ) ) ;
#25188=VERTEX_POINT ( 'NONE', #29455 ) ;
#25199=CARTESIAN_POINT ( 'NONE',  ( 53.80287614962789178, -40.05525454449572464, 69.29271901957253021 ) ) ;
#25215=CARTESIAN_POINT ( 'NONE',  ( -19.85879968743109458, -2.055254544495720648, 67.01652747270929922 ) ) ;
#25229=VERTEX_POINT ( 'NONE', #35547 ) ;
#25234=ORIENTED_EDGE ( 'NONE', *, *, #3555, .F. ) ;
#25387=CARTESIAN_POINT ( 'NONE',  ( 53.80287614962789178, -40.05525454449572464, 69.29271901957253021 ) ) ;
#25398=CARTESIAN_POINT ( 'NONE',  ( 22.90854556226722138, -2.055254544495723756, -74.83297477053847047 ) ) ;
#25458=CARTESIAN_POINT ( 'NONE',  ( -91.96080130434583566, -12.05525454449572109, 14.45886780445738395 ) ) ;
#25518=DIRECTION ( 'NONE',  ( 1.000000000000000000, 0.000000000000000000, 0.000000000000000000 ) ) ;
#25536=CIRCLE ( 'NONE', #16457, 15.99999999999998934 ) ;
#25541=ORIENTED_EDGE ( 'NONE', *, *, #21175, .F. ) ;
#25544=ORIENTED_EDGE ( 'NONE', *, *, #15080, .F. ) ;
#25575=DIRECTION ( 'NONE',  ( -1.000000000000000000, 1.577021341797063787E-16, 0.000000000000000000 ) ) ;
#25586=AXIS2_PLACEMENT_3D ( 'NONE', #9907, #40429, #6629 ) ;
#25587=DIRECTION ( 'NONE',  ( 1.058513553088275437E-16, 1.000000000000000000, -8.813324511995299047E-17 ) ) ;
#25630=AXIS2_PLACEMENT_3D ( 'NONE', #22118, #35577, #15762 ) ;
#25633=ORIENTED_EDGE ( 'NONE', *, *, #4116, .F. ) ;
#25651=DIRECTION ( 'NONE',  ( -1.058513553088275437E-16, -1.000000000000000000, 8.813324511995299047E-17 ) ) ;
#25680=DIRECTION ( 'NONE',  ( -1.058513553088275437E-16, -1.000000000000000000, 8.813324511995299047E-17 ) ) ;
#25733=CARTESIAN_POINT ( 'NONE',  ( -91.96080130434580724, -12.05525454449571043, 14.45886780445738218 ) ) ;
#25735=EDGE_CURVE ( 'NONE', #15816, #21731, #5760, .T. ) ;
#25750=ORIENTED_EDGE ( 'NONE', *, *, #9336, .T. ) ;
#25758=DIRECTION ( 'NONE',  ( 1.000000000000000000, -3.469446951953616038E-17, 0.000000000000000000 ) ) ;
#25799=CIRCLE ( 'NONE', #43163, 10.99999999999999645 ) ;
#25819=CARTESIAN_POINT ( 'NONE',  ( -135.4416936590755540, -2.055254544495720648, -102.7350398871816424 ) ) ;
#25828=AXIS2_PLACEMENT_3D ( 'NONE', #32218, #42229, #39171 ) ;
#25840=CARTESIAN_POINT ( 'NONE',  ( -102.9608013043458072, -34.05525454449571043, 14.45886780445738218 ) ) ;
#25887=AXIS2_PLACEMENT_3D ( 'NONE', #16052, #29558, #5768 ) ;
#25911=EDGE_CURVE ( 'NONE', #6283, #19076, #10399, .T. ) ;
#25954=EDGE_LOOP ( 'NONE', ( #21147, #31997, #28854, #530 ) ) ;
#26018=CARTESIAN_POINT ( 'NONE',  ( 22.90854556226710415, -35.35525454449573601, -74.83297477053821467 ) ) ;
#26074=DIRECTION ( 'NONE',  ( -3.009274222672345096E-17, -1.000000000000000000, 2.455023325076454960E-18 ) ) ;
#26109=CARTESIAN_POINT ( 'NONE',  ( 22.90854556226710415, -34.05525454449573175, -74.83297477053821467 ) ) ;
#26121=ORIENTED_EDGE ( 'NONE', *, *, #29652, .F. ) ;
#26131=EDGE_LOOP ( 'NONE', ( #31485, #3142, #32721, #21869 ) ) ;
#26140=CARTESIAN_POINT ( 'NONE',  ( 42.80287614962790599, -14.05525454449571932, 69.29271901957253021 ) ) ;
#26173=CARTESIAN_POINT ( 'NONE',  ( 33.90854556226734218, -40.05525454449572464, -74.83297477053821467 ) ) ;
#26189=AXIS2_PLACEMENT_3D ( 'NONE', #18668, #15157, #4645 ) ;
#26253=AXIS2_PLACEMENT_3D ( 'NONE', #25075, #24626, #5154 ) ;
#26284=EDGE_LOOP ( 'NONE', ( #38662, #32751, #14907, #2061 ) ) ;
#26289=FACE_OUTER_BOUND ( 'NONE', #40344, .T. ) ;
#26357=CARTESIAN_POINT ( 'NONE',  ( 12.40854556226731198, -35.35525454449573601, -74.83297477053802993 ) ) ;
#26430=EDGE_LOOP ( 'NONE', ( #23422, #1306 ) ) ;
#26504=CARTESIAN_POINT ( 'NONE',  ( 42.80287614962796994, -2.055254544495723756, 69.29271901957280022 ) ) ;
#26597=DIRECTION ( 'NONE',  ( -1.000000000000000000, 3.009274222672345096E-17, 0.000000000000000000 ) ) ;
#26613=FACE_BOUND ( 'NONE', #15333, .T. ) ;
#26647=EDGE_CURVE ( 'NONE', #36577, #37926, #1673, .T. ) ;
#26686=CIRCLE ( 'NONE', #32252, 16.00000000000023448 ) ;
#26721=APPLICATION_CONTEXT ( 'automotive_design' ) ;
#26722=VERTEX_POINT ( 'NONE', #10014 ) ;
#26728=EDGE_CURVE ( 'NONE', #19290, #1072, #9159, .T. ) ;
#26734=EDGE_LOOP ( 'NONE', ( #3534, #5968, #31099, #13700 ) ) ;
#26736=CARTESIAN_POINT ( 'NONE',  ( 22.90854556226722138, -2.055254544495723756, -74.83297477053847047 ) ) ;
#26765=CARTESIAN_POINT ( 'NONE',  ( 38.90854556226734218, -14.05525454449573175, -74.83297477053821467 ) ) ;
#26780=AXIS2_PLACEMENT_3D ( 'NONE', #16590, #29888, #26597 ) ;
#26781=ADVANCED_FACE ( 'NONE', ( #36406 ), #32287, .T. ) ;
#26823=EDGE_LOOP ( 'NONE', ( #17758, #8116 ) ) ;
#26879=EDGE_LOOP ( 'NONE', ( #13250, #24005 ) ) ;
#26886=DIRECTION ( 'NONE',  ( 3.009274222672345096E-17, 1.000000000000000000, -2.455023325076454960E-18 ) ) ;
#26889=VECTOR ( 'NONE', #13227, 1000.000000000000000 ) ;
#26893=ORIENTED_EDGE ( 'NONE', *, *, #8320, .F. ) ;
#26896=LINE ( 'NONE', #23651, #20380 ) ;
#26942=CIRCLE ( 'NONE', #17226, 10.49999999999999467 ) ;
#26970=DIRECTION ( 'NONE',  ( -1.000000000000000000, 0.000000000000000000, 0.000000000000000000 ) ) ;
#26974=ORIENTED_EDGE ( 'NONE', *, *, #26647, .F. ) ;
#26983=CARTESIAN_POINT ( 'NONE',  ( 38.90854556226734218, -12.05525454449572464, -74.83297477053821467 ) ) ;
#27035=SURFACE_SIDE_STYLE ('',( #20727 ) ) ;
#27055=LINE ( 'NONE', #20104, #22541 ) ;
#27058=EDGE_CURVE ( 'NONE', #1072, #41904, #9364, .T. ) ;
#27075=ADVANCED_FACE ( 'NONE', ( #41183 ), #12197, .T. ) ;
#27084=VERTEX_POINT ( 'NONE', #37919 ) ;
#27126=DIRECTION ( 'NONE',  ( 3.009274222672345096E-17, 1.000000000000000000, -2.455023325076454960E-18 ) ) ;
#27159=CIRCLE ( 'NONE', #18912, 10.99999999999998934 ) ;
#27163=AXIS2_PLACEMENT_3D ( 'NONE', #38698, #22178, #23026 ) ;
#27170=( NAMED_UNIT ( * ) SI_UNIT ( $, .STERADIAN. ) SOLID_ANGLE_UNIT ( ) );
#27178=EDGE_CURVE ( 'NONE', #9970, #41689, #15686, .T. ) ;
#27184=EDGE_CURVE ( 'NONE', #39162, #5150, #17068, .T. ) ;
#27222=VERTEX_POINT ( 'NONE', #29413 ) ;
#27225=LINE ( 'NONE', #1003, #38792 ) ;
#27238=EDGE_LOOP ( 'NONE', ( #42815, #9356, #27621, #17328 ) ) ;
#27241=( NAMED_UNIT ( * ) PLANE_ANGLE_UNIT ( ) SI_UNIT ( $, .RADIAN. ) );
#27247=AXIS2_PLACEMENT_3D ( 'NONE', #29986, #40615, #6832 ) ;
#27276=AXIS2_PLACEMENT_3D ( 'NONE', #26109, #12797, #42223 ) ;
#27299=CARTESIAN_POINT ( 'NONE',  ( 31.80287614962791665, -40.05525454449572464, 69.29271901957253021 ) ) ;
#27314=EDGE_CURVE ( 'NONE', #22843, #34135, #16333, .T. ) ;
#27353=FACE_OUTER_BOUND ( 'NONE', #31525, .T. ) ;
#27357=EDGE_LOOP ( 'NONE', ( #22388, #32621, #16481, #28878 ) ) ;
#27400=DIRECTION ( 'NONE',  ( 3.009274222672345096E-17, 1.000000000000000000, -2.455023325076455345E-18 ) ) ;
#27403=ORIENTED_EDGE ( 'NONE', *, *, #17227, .F. ) ;
#27412=DIRECTION ( 'NONE',  ( -3.009274222672345096E-17, -1.000000000000000000, 2.455023325076454960E-18 ) ) ;
#27416=EDGE_CURVE ( 'NONE', #16411, #9970, #41437, .T. ) ;
#27428=CARTESIAN_POINT ( 'NONE',  ( -80.96080130434580724, -40.05525454449572464, 14.45886780445738395 ) ) ;
#27450=VECTOR ( 'NONE', #16160, 1000.000000000000000 ) ;
#27466=AXIS2_PLACEMENT_3D ( 'NONE', #9265, #25680, #35456 ) ;
#27501=DIRECTION ( 'NONE',  ( 1.000000000000000000, -3.035766082959412415E-17, 0.000000000000000000 ) ) ;
#27531=LINE ( 'NONE', #39987, #7924 ) ;
#27545=CARTESIAN_POINT ( 'NONE',  ( 26.85238513915532721, -2.055254544495723756, 88.54322126041917329 ) ) ;
#27558=EDGE_LOOP ( 'NONE', ( #33591, #14169, #33618, #17946 ) ) ;
#27563=DIRECTION ( 'NONE',  ( -1.058513553088275437E-16, -1.000000000000000000, 8.813324511995299047E-17 ) ) ;
#27603=VECTOR ( 'NONE', #16777, 1000.000000000000000 ) ;
#27613=AXIS2_PLACEMENT_3D ( 'NONE', #13576, #36663, #4359 ) ;
#27621=ORIENTED_EDGE ( 'NONE', *, *, #28389, .T. ) ;
#27626=CARTESIAN_POINT ( 'NONE',  ( -102.0670434220619427, -2.055254544495720648, 139.0496534599708980 ) ) ;
#27669=CIRCLE ( 'NONE', #26253, 10.99999999999998934 ) ;
#27703=DIRECTION ( 'NONE',  ( -1.000000000000000000, 1.084202172485488534E-16, 0.000000000000000000 ) ) ;
#27717=FACE_OUTER_BOUND ( 'NONE', #14799, .T. ) ;
#27755=EDGE_CURVE ( 'NONE', #37926, #36577, #2428, .T. ) ;
#27791=FACE_OUTER_BOUND ( 'NONE', #13621, .T. ) ;
#27827=CARTESIAN_POINT ( 'NONE',  ( 22.90854556226710415, -40.05525454449572464, -74.83297477053821467 ) ) ;
#27835=CARTESIAN_POINT ( 'NONE',  ( -91.96080130434573618, -35.35525454449571470, 14.45886780445633946 ) ) ;
#27868=CARTESIAN_POINT ( 'NONE',  ( -80.96080130434580724, -35.35525454449571470, 14.45886780445738395 ) ) ;
#27869=ORIENTED_EDGE ( 'NONE', *, *, #37480, .T. ) ;
#27875=EDGE_CURVE ( 'NONE', #33033, #32706, #37301, .T. ) ;
#27879=MANIFOLD_SOLID_BREP ( 'Boss-Extrude4', #35842 ) ;
#27882=CARTESIAN_POINT ( 'NONE',  ( 2.339412683011424576, -2.055254544495723756, -89.04250581823735899 ) ) ;
#27991=DIRECTION ( 'NONE',  ( -1.058513553088275437E-16, -1.000000000000000000, 8.813324511995299047E-17 ) ) ;
#27998=DIRECTION ( 'NONE',  ( -1.000000000000000000, 0.000000000000000000, 0.000000000000000000 ) ) ;
#28013=DIRECTION ( 'NONE',  ( 3.009274222672345096E-17, 1.000000000000000000, -2.455023325076454960E-18 ) ) ;
#28034=ADVANCED_FACE ( 'NONE', ( #14953 ), #1168, .T. ) ;
#28044=ORIENTED_EDGE ( 'NONE', *, *, #41032, .F. ) ;
#28064=ORIENTED_EDGE ( 'NONE', *, *, #42956, .F. ) ;
#28176=VERTEX_POINT ( 'NONE', #25840 ) ;
#28179=FACE_OUTER_BOUND ( 'NONE', #27238, .T. ) ;
#28207=DIRECTION ( 'NONE',  ( -3.009274222672345096E-17, -1.000000000000000000, 2.455023325076455345E-18 ) ) ;
#28211=CYLINDRICAL_SURFACE ( 'NONE', #35395, 24.99999999999999289 ) ;
#28213=FACE_OUTER_BOUND ( 'NONE', #8508, .T. ) ;
#28229=DIRECTION ( 'NONE',  ( -1.000000000000000000, 0.000000000000000000, 0.000000000000000000 ) ) ;
#28305=VECTOR ( 'NONE', #38121, 1000.000000000000000 ) ;
#28309=EDGE_LOOP ( 'NONE', ( #21066, #6692 ) ) ;
#28330=ORIENTED_EDGE ( 'NONE', *, *, #7567, .F. ) ;
#28332=FACE_OUTER_BOUND ( 'NONE', #36431, .T. ) ;
#28389=EDGE_CURVE ( 'NONE', #23370, #34135, #17272, .T. ) ;
#28391=CYLINDRICAL_SURFACE ( 'NONE', #37196, 65.00000000000000000 ) ;
#28417=ORIENTED_EDGE ( 'NONE', *, *, #87, .T. ) ;
#28451=DIRECTION ( 'NONE',  ( -3.009274222672345096E-17, -1.000000000000000000, 2.455023325076454960E-18 ) ) ;
#28455=ADVANCED_FACE ( 'NONE', ( #17694, #14406, #27717 ), #28790, .T. ) ;
#28465=CIRCLE ( 'NONE', #15242, 100.0000000000000711 ) ;
#28510=VERTEX_POINT ( 'NONE', #35517 ) ;
#28544=EDGE_LOOP ( 'NONE', ( #39450, #25089 ) ) ;
#28555=CARTESIAN_POINT ( 'NONE',  ( 42.80287614962790599, -12.05525454449572464, 69.29271901957253021 ) ) ;
#28556=ORIENTED_EDGE ( 'NONE', *, *, #11522, .T. ) ;
#28571=FACE_OUTER_BOUND ( 'NONE', #41440, .T. ) ;
#28624=EDGE_CURVE ( 'NONE', #30653, #6921, #22913, .T. ) ;
#28626=CARTESIAN_POINT ( 'NONE',  ( -24.74979319748359785, -2.055254544495722868, 2.972870684497277427 ) ) ;
#28649=DIRECTION ( 'NONE',  ( 1.058513553088275437E-16, 1.000000000000000000, -8.813324511995299047E-17 ) ) ;
#28654=CARTESIAN_POINT ( 'NONE',  ( 26.80287614962791309, -12.05525454449572464, 69.29271901957253021 ) ) ;
#28669=EDGE_LOOP ( 'NONE', ( #30503, #30699, #18261, #32498 ) ) ;
#28713=EDGE_CURVE ( 'NONE', #24613, #15816, #27225, .T. ) ;
#28790=PLANE ( 'NONE',  #41535 ) ;
#28851=ORIENTED_EDGE ( 'NONE', *, *, #32284, .F. ) ;
#28854=ORIENTED_EDGE ( 'NONE', *, *, #24742, .F. ) ;
#28878=ORIENTED_EDGE ( 'NONE', *, *, #3936, .F. ) ;
#28920=CARTESIAN_POINT ( 'NONE',  ( 42.80287614962790599, -12.05525454449571932, 69.29271901957253021 ) ) ;
#28924=DIRECTION ( 'NONE',  ( 1.000000000000000000, -3.035766082959412415E-17, 0.000000000000000000 ) ) ;
#28996=ORIENTED_EDGE ( 'NONE', *, *, #43033, .F. ) ;
#29019=CARTESIAN_POINT ( 'NONE',  ( 155.7547826636224499, -12.05525454449572820, 15.74958860255448734 ) ) ;
#29078=CARTESIAN_POINT ( 'NONE',  ( 42.80287614962796994, -2.055254544495723756, 69.29271901957280022 ) ) ;
#29101=AXIS2_PLACEMENT_3D ( 'NONE', #33045, #29581, #19567 ) ;
#29111=DIRECTION ( 'NONE',  ( -3.009274222672345096E-17, -1.000000000000000000, 2.455023325076454960E-18 ) ) ;
#29166=ADVANCED_BREP_SHAPE_REPRESENTATION ( '', ( #27879, #13552 ), #21242 ) ;
#29183=CYLINDRICAL_SURFACE ( 'NONE', #39198, 11.00000000000000000 ) ;
#29205=DIRECTION ( 'NONE',  ( 3.009274222672345096E-17, 1.000000000000000000, -2.455023325076454960E-18 ) ) ;
#29252=ADVANCED_FACE ( 'NONE', ( #5101, #4675 ), #11242, .F. ) ;
#29258=DIRECTION ( 'NONE',  ( 3.009274222672345096E-17, 1.000000000000000000, -2.455023325076455345E-18 ) ) ;
#29295=EDGE_CURVE ( 'NONE', #3091, #6921, #24240, .T. ) ;
#29362=EDGE_CURVE ( 'NONE', #30346, #38270, #21312, .T. ) ;
#29379=DIRECTION ( 'NONE',  ( -1.058513553088275437E-16, -1.000000000000000000, 8.813324511995299047E-17 ) ) ;
#29389=CARTESIAN_POINT ( 'NONE',  ( 65.39325745242679488, -2.055254544495723756, 58.58409293616905700 ) ) ;
#29413=CARTESIAN_POINT ( 'NONE',  ( 53.80287614962789178, -14.05525454449572109, 69.29271901957253021 ) ) ;
#29424=VECTOR ( 'NONE', #29111, 1000.000000000000000 ) ;
#29430=DIRECTION ( 'NONE',  ( 3.009274222672345096E-17, 1.000000000000000000, -2.455023325076455345E-18 ) ) ;
#29455=CARTESIAN_POINT ( 'NONE',  ( 6.908545562266867002, -14.05525454449572820, -74.83297477053821467 ) ) ;
#29482=CARTESIAN_POINT ( 'NONE',  ( -8.749793197483594298, -2.055254544495723756, 2.972870684497274762 ) ) ;
#29489=CYLINDRICAL_SURFACE ( 'NONE', #30675, 100.0000000000000711 ) ;
#29508=DIRECTION ( 'NONE',  ( 3.009274222672345096E-17, 1.000000000000000000, -2.455023325076454960E-18 ) ) ;
#29550=CARTESIAN_POINT ( 'NONE',  ( 42.80287614962723808, -35.35525454449572180, 69.29271901957299917 ) ) ;
#29557=ORIENTED_EDGE ( 'NONE', *, *, #6683, .F. ) ;
#29558=DIRECTION ( 'NONE',  ( -3.009274222672345096E-17, -1.000000000000000000, 2.455023325076454960E-18 ) ) ;
#29566=EDGE_CURVE ( 'NONE', #9805, #12272, #30508, .T. ) ;
#29581=DIRECTION ( 'NONE',  ( 1.058513553088275437E-16, 1.000000000000000000, -8.813324511995299047E-17 ) ) ;
#29652=EDGE_CURVE ( 'NONE', #8193, #18529, #3299, .T. ) ;
#29673=ORIENTED_EDGE ( 'NONE', *, *, #15315, .T. ) ;
#29675=DIRECTION ( 'NONE',  ( -1.000000000000000000, 0.000000000000000000, 0.000000000000000000 ) ) ;
#29714=FACE_OUTER_BOUND ( 'NONE', #39880, .T. ) ;
#29723=VECTOR ( 'NONE', #4544, 1000.000000000000000 ) ;
#29744=DIRECTION ( 'NONE',  ( 1.000000000000000000, -3.469446951953614189E-17, 0.000000000000000000 ) ) ;
#29764=ADVANCED_FACE ( 'NONE', ( #31901 ), #8115, .T. ) ;
#29776=ORIENTED_EDGE ( 'NONE', *, *, #10844, .F. ) ;
#29888=DIRECTION ( 'NONE',  ( 3.009274222672345096E-17, 1.000000000000000000, -2.455023325076454960E-18 ) ) ;
#29904=CARTESIAN_POINT ( 'NONE',  ( -45.51113419504475388, -2.055254544495720648, 56.57887602028989704 ) ) ;
#29928=FACE_OUTER_BOUND ( 'NONE', #39325, .T. ) ;
#29931=CARTESIAN_POINT ( 'NONE',  ( -19.85879968743109458, -12.05525454449572109, 67.01652747270929922 ) ) ;
#29960=ORIENTED_EDGE ( 'NONE', *, *, #14876, .F. ) ;
#29974=CARTESIAN_POINT ( 'NONE',  ( 52.26814377733353467, -12.05525454449572464, -19.42827587850796434 ) ) ;
#29986=CARTESIAN_POINT ( 'NONE',  ( 42.80287614962790599, -40.05525454449572464, 69.29271901957253021 ) ) ;
#30077=VERTEX_POINT ( 'NONE', #185 ) ;
#30082=ORIENTED_EDGE ( 'NONE', *, *, #30198, .F. ) ;
#30150=EDGE_CURVE ( 'NONE', #34172, #8500, #16638, .T. ) ;
#30198=EDGE_CURVE ( 'NONE', #24613, #30077, #12357, .T. ) ;
#30268=ADVANCED_FACE ( 'NONE', ( #34453 ), #31208, .F. ) ;
#30332=CARTESIAN_POINT ( 'NONE',  ( -26.14979319748359643, 5.944745455504278020, 2.972870684497277427 ) ) ;
#30346=VERTEX_POINT ( 'NONE', #39374 ) ;
#30378=CARTESIAN_POINT ( 'NONE',  ( 47.90854556226721428, -2.055254544495724645, -74.83297477053847047 ) ) ;
#30422=ORIENTED_EDGE ( 'NONE', *, *, #26647, .T. ) ;
#30460=CYLINDRICAL_SURFACE ( 'NONE', #32096, 10.49999999999998934 ) ;
#30473=VECTOR ( 'NONE', #17812, 1000.000000000000000 ) ;
#30503=ORIENTED_EDGE ( 'NONE', *, *, #29566, .T. ) ;
#30508=CIRCLE ( 'NONE', #15216, 65.00000000000000000 ) ;
#30526=CARTESIAN_POINT ( 'NONE',  ( 42.80287614962723808, -34.05525454449571754, 69.29271901957299917 ) ) ;
#30567=AXIS2_PLACEMENT_3D ( 'NONE', #32784, #36257, #12737 ) ;
#30653=VERTEX_POINT ( 'NONE', #14968 ) ;
#30666=CARTESIAN_POINT ( 'NONE',  ( 31.80287614962791665, -35.35525454449572180, 69.29271901957253021 ) ) ;
#30675=AXIS2_PLACEMENT_3D ( 'NONE', #39493, #6133, #15557 ) ;
#30699=ORIENTED_EDGE ( 'NONE', *, *, #40112, .F. ) ;
#30702=ORIENTED_EDGE ( 'NONE', *, *, #17048, .F. ) ;
#30735=CARTESIAN_POINT ( 'NONE',  ( -8.749793197483594298, -2.055254544495723756, 2.972870684497274762 ) ) ;
#30748=CARTESIAN_POINT ( 'NONE',  ( -91.96080130434580724, -14.05525454449571043, 14.45886780445738218 ) ) ;
#30780=ORIENTED_EDGE ( 'NONE', *, *, #19578, .F. ) ;
#30808=DIRECTION ( 'NONE',  ( -1.000000000000000000, 0.000000000000000000, 0.000000000000000000 ) ) ;
#30823=ADVANCED_FACE ( 'NONE', ( #32369 ), #42599, .T. ) ;
#30832=ORIENTED_EDGE ( 'NONE', *, *, #38643, .T. ) ;
#30906=DIRECTION ( 'NONE',  ( -1.000000000000000000, 0.000000000000000000, 0.000000000000000000 ) ) ;
#30979=CARTESIAN_POINT ( 'NONE',  ( 42.80287614962723808, -35.35525454449572180, 69.29271901957299917 ) ) ;
#30994=AXIS2_PLACEMENT_3D ( 'NONE', #7116, #20916, #33524 ) ;
#31017=AXIS2_PLACEMENT_3D ( 'NONE', #18429, #28013, #41273 ) ;
#31025=DIRECTION ( 'NONE',  ( -1.058513553088275437E-16, -1.000000000000000000, 8.813324511995299047E-17 ) ) ;
#31049=AXIS2_PLACEMENT_3D ( 'NONE', #13800, #20143, #33401 ) ;
#31079=DIRECTION ( 'NONE',  ( 1.000000000000000000, 0.000000000000000000, 0.000000000000000000 ) ) ;
#31096=VERTEX_POINT ( 'NONE', #33651 ) ;
#31097=DIRECTION ( 'NONE',  ( 1.000000000000000000, 0.000000000000000000, 0.000000000000000000 ) ) ;
#31099=ORIENTED_EDGE ( 'NONE', *, *, #41032, .T. ) ;
#31101=ORIENTED_EDGE ( 'NONE', *, *, #35137, .F. ) ;
#31166=DIRECTION ( 'NONE',  ( -1.000000000000000000, 0.000000000000000000, 0.000000000000000000 ) ) ;
#31168=CYLINDRICAL_SURFACE ( 'NONE', #40448, 10.49999999999999112 ) ;
#31170=EDGE_CURVE ( 'NONE', #37998, #8193, #40563, .T. ) ;
#31179=ORIENTED_EDGE ( 'NONE', *, *, #23388, .F. ) ;
#31208=CYLINDRICAL_SURFACE ( 'NONE', #38789, 100.0000000000000000 ) ;
#31234=EDGE_LOOP ( 'NONE', ( #4021, #19828 ) ) ;
#31268=DIRECTION ( 'NONE',  ( -1.000000000000000000, 0.000000000000000000, 0.000000000000000000 ) ) ;
#31338=EDGE_CURVE ( 'NONE', #17494, #19198, #11474, .T. ) ;
#31381=DIRECTION ( 'NONE',  ( 3.009274222672345096E-17, 1.000000000000000000, -2.455023325076454960E-18 ) ) ;
#31407=ADVANCED_FACE ( 'NONE', ( #39015 ), #28391, .T. ) ;
#31425=AXIS2_PLACEMENT_3D ( 'NONE', #39869, #23140, #13092 ) ;
#31431=ORIENTED_EDGE ( 'NONE', *, *, #38096, .T. ) ;
#31477=CARTESIAN_POINT ( 'NONE',  ( 32.30287614962725229, -34.05525454449571754, 69.29271901957299917 ) ) ;
#31485=ORIENTED_EDGE ( 'NONE', *, *, #191, .F. ) ;
#31509=EDGE_LOOP ( 'NONE', ( #24627, #36052, #14212, #11081 ) ) ;
#31514=ADVANCED_FACE ( 'NONE', ( #33124, #16141, #3212, #22706 ), #33351, .F. ) ;
#31525=EDGE_LOOP ( 'NONE', ( #23603, #27403, #38303, #9957 ) ) ;
#31527=CARTESIAN_POINT ( 'NONE',  ( 42.80287614962790599, -40.05525454449572464, 69.29271901957253021 ) ) ;
#31621=AXIS2_PLACEMENT_3D ( 'NONE', #5684, #25587, #38843 ) ;
#31664=COLOUR_RGB ( '', 0.66274510, 0.83137255, 0.94901961) ;
#31705=AXIS2_PLACEMENT_3D ( 'NONE', #29078, #12282, #42348 ) ;
#31714=ORIENTED_EDGE ( 'NONE', *, *, #683, .F. ) ;
#31737=CIRCLE ( 'NONE', #12926, 10.49999999999999467 ) ;
#31768=DIRECTION ( 'NONE',  ( 3.009274222672345096E-17, 1.000000000000000000, -2.455023325076455345E-18 ) ) ;
#31769=CIRCLE ( 'NONE', #26189, 15.99999999999998579 ) ;
#31827=EDGE_LOOP ( 'NONE', ( #6935, #15130 ) ) ;
#31834=CIRCLE ( 'NONE', #20026, 11.00000000000023803 ) ;
#31849=AXIS2_PLACEMENT_3D ( 'NONE', #33129, #36388, #16146 ) ;
#31901=FACE_OUTER_BOUND ( 'NONE', #31988, .T. ) ;
#31945=DIRECTION ( 'NONE',  ( 2.731800627175558911E-17, 1.000000000000000000, -3.170996607629411740E-18 ) ) ;
#31986=LINE ( 'NONE', #22408, #19791 ) ;
#31988=EDGE_LOOP ( 'NONE', ( #42009, #28556, #41684, #30702 ) ) ;
#31997=ORIENTED_EDGE ( 'NONE', *, *, #736, .F. ) ;
#32005=EDGE_CURVE ( 'NONE', #26722, #6283, #41430, .T. ) ;
#32014=VECTOR ( 'NONE', #3319, 1000.000000000000000 ) ;
#32037=ORIENTED_EDGE ( 'NONE', *, *, #21847, .T. ) ;
#32084=EDGE_CURVE ( 'NONE', #26722, #31096, #34751, .T. ) ;
#32096=AXIS2_PLACEMENT_3D ( 'NONE', #13457, #16955, #26970 ) ;
#32107=DIRECTION ( 'NONE',  ( -3.009274222672345096E-17, -1.000000000000000000, 2.455023325076454960E-18 ) ) ;
#32159=FACE_BOUND ( 'NONE', #15517, .T. ) ;
#32181=ORIENTED_EDGE ( 'NONE', *, *, #191, .T. ) ;
#32194=AXIS2_PLACEMENT_3D ( 'NONE', #7951, #34569, #31097 ) ;
#32198=DIRECTION ( 'NONE',  ( 1.000000000000000000, 0.000000000000000000, 0.000000000000000000 ) ) ;
#32217=EDGE_CURVE ( 'NONE', #12532, #16411, #20580, .T. ) ;
#32218=CARTESIAN_POINT ( 'NONE',  ( -24.74979319748359785, 5.944745455504278020, 2.972870684497277427 ) ) ;
#32252=AXIS2_PLACEMENT_3D ( 'NONE', #40746, #10898, #27703 ) ;
#32264=ORIENTED_EDGE ( 'NONE', *, *, #32217, .F. ) ;
#32284=EDGE_CURVE ( 'NONE', #19290, #39162, #34492, .T. ) ;
#32287=PLANE ( 'NONE',  #10019 ) ;
#32322=DIRECTION ( 'NONE',  ( -1.000000000000000000, 1.084202172485505174E-16, 0.000000000000000000 ) ) ;
#32329=CARTESIAN_POINT ( 'NONE',  ( -91.96080130434573618, -34.05525454449571043, 14.45886780445633946 ) ) ;
#32369=FACE_OUTER_BOUND ( 'NONE', #6457, .T. ) ;
#32374=ORIENTED_EDGE ( 'NONE', *, *, #31338, .F. ) ;
#32391=ADVANCED_FACE ( 'NONE', ( #19914, #16863 ), #10050, .T. ) ;
#32479=AXIS2_PLACEMENT_3D ( 'NONE', #25458, #8618, #11720 ) ;
#32498=ORIENTED_EDGE ( 'NONE', *, *, #36160, .T. ) ;
#32506=DIRECTION ( 'NONE',  ( -1.000000000000000000, 3.009274222672345096E-17, 0.000000000000000000 ) ) ;
#32515=AXIS2_PLACEMENT_3D ( 'NONE', #28920, #9047, #36288 ) ;
#32534=ADVANCED_FACE ( 'NONE', ( #29714 ), #13145, .T. ) ;
#32539=EDGE_LOOP ( 'NONE', ( #32264, #15372, #40155, #28330 ) ) ;
#32584=FACE_OUTER_BOUND ( 'NONE', #7144, .T. ) ;
#32616=CYLINDRICAL_SURFACE ( 'NONE', #42258, 10.49999999999999112 ) ;
#32621=ORIENTED_EDGE ( 'NONE', *, *, #23810, .T. ) ;
#32629=DIRECTION ( 'NONE',  ( 1.000000000000000000, 0.000000000000000000, 0.000000000000000000 ) ) ;
#32682=CARTESIAN_POINT ( 'NONE',  ( 42.80287614962723808, -35.35525454449572180, 69.29271901957299917 ) ) ;
#32706=VERTEX_POINT ( 'NONE', #42299 ) ;
#32721=ORIENTED_EDGE ( 'NONE', *, *, #4012, .F. ) ;
#32751=ORIENTED_EDGE ( 'NONE', *, *, #14557, .T. ) ;
#32754=DIRECTION ( 'NONE',  ( -1.000000000000000000, 3.035766082959412415E-17, 0.000000000000000000 ) ) ;
#32777=ORIENTED_EDGE ( 'NONE', *, *, #15852, .T. ) ;
#32783=ORIENTED_EDGE ( 'NONE', *, *, #34748, .F. ) ;
#32784=CARTESIAN_POINT ( 'NONE',  ( -8.749793197483592522, 117.9447454555042754, 2.972870684497274762 ) ) ;
#32802=CIRCLE ( 'NONE', #31425, 10.99999999999999645 ) ;
#32810=AXIS2_PLACEMENT_3D ( 'NONE', #6301, #32917, #23785 ) ;
#32846=CARTESIAN_POINT ( 'NONE',  ( -8.749793197483596074, -2.055254544495723312, 2.972870684497275207 ) ) ;
#32871=DIRECTION ( 'NONE',  ( 1.000000000000000000, 0.000000000000000000, 0.000000000000000000 ) ) ;
#32917=DIRECTION ( 'NONE',  ( 3.009274222672345096E-17, 1.000000000000000000, -2.455023325076455345E-18 ) ) ;
#32925=CIRCLE ( 'NONE', #861, 99.99999999999994316 ) ;
#32998=FACE_BOUND ( 'NONE', #21525, .T. ) ;
#33003=VECTOR ( 'NONE', #16624, 1000.000000000000000 ) ;
#33009=CYLINDRICAL_SURFACE ( 'NONE', #27247, 10.99999999999998934 ) ;
#33033=VERTEX_POINT ( 'NONE', #11110 ) ;
#33034=VECTOR ( 'NONE', #22673, 1000.000000000000000 ) ;
#33045=CARTESIAN_POINT ( 'NONE',  ( 42.80287614962790599, -14.05525454449571932, 69.29271901957253021 ) ) ;
#33124=FACE_BOUND ( 'NONE', #23311, .T. ) ;
#33129=CARTESIAN_POINT ( 'NONE',  ( -91.96080130434580724, -40.05525454449572464, 14.45886780445738218 ) ) ;
#33135=CYLINDRICAL_SURFACE ( 'NONE', #32810, 10.99999999999999645 ) ;
#33152=CIRCLE ( 'NONE', #14368, 64.99999999999997158 ) ;
#33161=CARTESIAN_POINT ( 'NONE',  ( -107.9608013043457930, -12.05525454449571043, 14.45886780445738395 ) ) ;
#33172=PLANE ( 'NONE',  #17261 ) ;
#33245=PRODUCT ( 'Planetary Gear Carrier Assembly', 'Planetary Gear Carrier Assembly', '', ( #22722 ) ) ;
#33266=CARTESIAN_POINT ( 'NONE',  ( 22.90854556226710415, -40.05525454449572464, -74.83297477053821467 ) ) ;
#33283=DIRECTION ( 'NONE',  ( 3.009274222672345096E-17, 1.000000000000000000, -2.455023325076454960E-18 ) ) ;
#33346=AXIS2_PLACEMENT_3D ( 'NONE', #34456, #37300, #27501 ) ;
#33348=VECTOR ( 'NONE', #20078, 1000.000000000000000 ) ;
#33351=PLANE ( 'NONE',  #26780 ) ;
#33364=DIRECTION ( 'NONE',  ( 3.009274222672345096E-17, 1.000000000000000000, -2.455023325076455345E-18 ) ) ;
#33370=EDGE_LOOP ( 'NONE', ( #6610, #29557, #20084, #4278, #28044, #13833, #31714, #14023, #32374, #17502, #10684, #24200, #33626, #15420, #31179 ) ) ;
#33380=LINE ( 'NONE', #7179, #35540 ) ;
#33385=CARTESIAN_POINT ( 'NONE',  ( 42.80287614962790599, -35.35525454449572180, 69.29271901957253021 ) ) ;
#33392=ORIENTED_EDGE ( 'NONE', *, *, #7080, .T. ) ;
#33401=DIRECTION ( 'NONE',  ( 1.000000000000000000, -1.058513553088275437E-16, 0.000000000000000000 ) ) ;
#33404=CARTESIAN_POINT ( 'NONE',  ( 22.90854556226722138, -2.055254544495723756, -74.83297477053847047 ) ) ;
#33409=CARTESIAN_POINT ( 'NONE',  ( 47.55521504368574881, -12.05525454449572464, -70.64469547305695585 ) ) ;
#33423=ORIENTED_EDGE ( 'NONE', *, *, #27416, .F. ) ;
#33428=AXIS2_PLACEMENT_3D ( 'NONE', #36876, #39914, #36650 ) ;
#33446=VERTEX_POINT ( 'NONE', #39183 ) ;
#33512=CIRCLE ( 'NONE', #17515, 10.49999999999999467 ) ;
#33524=DIRECTION ( 'NONE',  ( -1.000000000000000000, 3.035766082959412415E-17, 0.000000000000000000 ) ) ;
#33560=DIRECTION ( 'NONE',  ( -1.000000000000000000, 3.336006684570783348E-17, 0.000000000000000000 ) ) ;
#33591=ORIENTED_EDGE ( 'NONE', *, *, #6606, .T. ) ;
#33618=ORIENTED_EDGE ( 'NONE', *, *, #10619, .T. ) ;
#33626=ORIENTED_EDGE ( 'NONE', *, *, #24244, .F. ) ;
#33651=CARTESIAN_POINT ( 'NONE',  ( -93.98204972788910538, -12.05525454449572109, 39.37702493556011518 ) ) ;
#33686=PRESENTATION_STYLE_ASSIGNMENT (( #521 ) ) ;
#33699=ORIENTED_EDGE ( 'NONE', *, *, #1684, .T. ) ;
#33754=CARTESIAN_POINT ( 'NONE',  ( 33.90854556226734218, -40.05525454449572464, -74.83297477053821467 ) ) ;
#33766=( LENGTH_UNIT ( ) NAMED_UNIT ( * ) SI_UNIT ( .MILLI., .METRE. ) );
#33827=DIRECTION ( 'NONE',  ( -3.009274222672345096E-17, -1.000000000000000000, 2.455023325076454960E-18 ) ) ;
#33898=ORIENTED_EDGE ( 'NONE', *, *, #29295, .T. ) ;
#33935=CYLINDRICAL_SURFACE ( 'NONE', #704, 10.99999999999998934 ) ;
#33942=AXIS2_PLACEMENT_3D ( 'NONE', #33385, #9821, #3898 ) ;
#33996=DIRECTION ( 'NONE',  ( 1.000000000000000000, 0.000000000000000000, 0.000000000000000000 ) ) ;
#34000=ORIENTED_EDGE ( 'NONE', *, *, #26728, .F. ) ;
#34028=DIRECTION ( 'NONE',  ( -3.009274222672345096E-17, -1.000000000000000000, 2.455023325076455345E-18 ) ) ;
#34135=VERTEX_POINT ( 'NONE', #14719 ) ;
#34165=EDGE_CURVE ( 'NONE', #32706, #33033, #31769, .T. ) ;
#34172=VERTEX_POINT ( 'NONE', #11430 ) ;
#34200=EDGE_LOOP ( 'NONE', ( #25544, #8057, #1048, #37041 ) ) ;
#34232=LINE ( 'NONE', #1054, #24996 ) ;
#34266=VECTOR ( 'NONE', #4340, 1000.000000000000000 ) ;
#34374=CARTESIAN_POINT ( 'NONE',  ( 58.80287614962789888, -12.05525454449572464, 69.29271901957253021 ) ) ;
#34404=CYLINDRICAL_SURFACE ( 'NONE', #19050, 11.00000000000000000 ) ;
#34443=FACE_OUTER_BOUND ( 'NONE', #16877, .T. ) ;
#34453=FACE_OUTER_BOUND ( 'NONE', #25954, .T. ) ;
#34454=EDGE_LOOP ( 'NONE', ( #30832, #8313 ) ) ;
#34456=CARTESIAN_POINT ( 'NONE',  ( -79.93711883401132923, -2.055254544495720648, -145.8806300090334673 ) ) ;
#34484=CARTESIAN_POINT ( 'NONE',  ( -91.96080130434580724, -12.05525454449572109, 14.45886780445738218 ) ) ;
#34486=ADVANCED_FACE ( 'NONE', ( #19202 ), #2562, .T. ) ;
#34492=CIRCLE ( 'NONE', #31705, 25.00000000000000000 ) ;
#34501=EDGE_LOOP ( 'NONE', ( #22639, #6015 ) ) ;
#34558=LINE ( 'NONE', #10799, #8227 ) ;
#34561=CARTESIAN_POINT ( 'NONE',  ( -19.74979319748359430, 117.9447454555042754, 2.972870684497276095 ) ) ;
#34569=DIRECTION ( 'NONE',  ( -3.009274222672345096E-17, -1.000000000000000000, 2.455023325076455345E-18 ) ) ;
#34600=VERTEX_POINT ( 'NONE', #3419 ) ;
#34671=DIRECTION ( 'NONE',  ( -3.009274222672345096E-17, -1.000000000000000000, 2.455023325076454960E-18 ) ) ;
#34673=DIRECTION ( 'NONE',  ( -1.000000000000000000, 0.000000000000000000, 0.000000000000000000 ) ) ;
#34738=CARTESIAN_POINT ( 'NONE',  ( -23.34979319748359927, 5.944745455504278020, 2.972870684497277427 ) ) ;
#34745=CYLINDRICAL_SURFACE ( 'NONE', #2055, 11.00000000000023448 ) ;
#34748=EDGE_CURVE ( 'NONE', #37926, #8001, #20710, .T. ) ;
#34751=LINE ( 'NONE', #14922, #40040 ) ;
#34754=DIRECTION ( 'NONE',  ( -1.000000000000000000, 0.000000000000000000, 0.000000000000000000 ) ) ;
#34800=DIRECTION ( 'NONE',  ( -1.058513553088275437E-16, -1.000000000000000000, 8.813324511995299047E-17 ) ) ;
#34849=EDGE_CURVE ( 'NONE', #27222, #19395, #27669, .T. ) ;
#34880=DIRECTION ( 'NONE',  ( -1.000000000000000000, 3.009274222672345096E-17, 0.000000000000000000 ) ) ;
#34930=EDGE_CURVE ( 'NONE', #13563, #8001, #31834, .T. ) ;
#35009=DIRECTION ( 'NONE',  ( 1.000000000000000000, -3.035766082959412415E-17, 0.000000000000000000 ) ) ;
#35121=CARTESIAN_POINT ( 'NONE',  ( 22.90854556226710415, -12.05525454449572997, -74.83297477053821467 ) ) ;
#35137=EDGE_CURVE ( 'NONE', #9970, #27084, #35333, .T. ) ;
#35280=VECTOR ( 'NONE', #31945, 1000.000000000000000 ) ;
#35284=CARTESIAN_POINT ( 'NONE',  ( 31.80287614962791665, -40.05525454449572464, 69.29271901957253021 ) ) ;
#35333=CIRCLE ( 'NONE', #4688, 24.99999999999998934 ) ;
#35359=DIRECTION ( 'NONE',  ( -1.000000000000000000, 0.000000000000000000, 0.000000000000000000 ) ) ;
#35363=FACE_OUTER_BOUND ( 'NONE', #34200, .T. ) ;
#35393=DIRECTION ( 'NONE',  ( 1.000000000000000000, -1.058513553088275437E-16, 0.000000000000000000 ) ) ;
#35395=AXIS2_PLACEMENT_3D ( 'NONE', #41044, #14250, #4618 ) ;
#35400=AXIS2_PLACEMENT_3D ( 'NONE', #21419, #34671, #4785 ) ;
#35421=DIRECTION ( 'NONE',  ( 2.932542530036133930E-17, 1.000000000000000000, -5.216001792149171863E-18 ) ) ;
#35456=DIRECTION ( 'NONE',  ( 1.000000000000000000, 0.000000000000000000, 0.000000000000000000 ) ) ;
#35463=CARTESIAN_POINT ( 'NONE',  ( -91.96080130434573618, -35.35525454449571470, 14.45886780445633946 ) ) ;
#35477=ORIENTED_EDGE ( 'NONE', *, *, #17716, .F. ) ;
#35486=ORIENTED_EDGE ( 'NONE', *, *, #982, .F. ) ;
#35512=ORIENTED_EDGE ( 'NONE', *, *, #12137, .T. ) ;
#35517=CARTESIAN_POINT ( 'NONE',  ( -19.85879968743109458, -2.055254544495720648, 67.01652747270929922 ) ) ;
#35528=CARTESIAN_POINT ( 'NONE',  ( -80.96080130434580724, -40.05525454449572464, 14.45886780445738395 ) ) ;
#35533=AXIS2_PLACEMENT_3D ( 'NONE', #10079, #39532, #12952 ) ;
#35540=VECTOR ( 'NONE', #16843, 1000.000000000000000 ) ;
#35547=CARTESIAN_POINT ( 'NONE',  ( -100.6569797752917879, -12.05525454449572109, -8.979913733870429127 ) ) ;
#35556=EDGE_LOOP ( 'NONE', ( #19908, #22726 ) ) ;
#35577=DIRECTION ( 'NONE',  ( 3.009274222672345096E-17, 1.000000000000000000, -2.455023325076454960E-18 ) ) ;
#35580=EDGE_LOOP ( 'NONE', ( #38483, #19871 ) ) ;
#35714=ADVANCED_FACE ( 'NONE', ( #7027 ), #20382, .T. ) ;
#35752=ORIENTED_EDGE ( 'NONE', *, *, #15189, .F. ) ;
#35795=DIRECTION ( 'NONE',  ( -1.058513553088275437E-16, -1.000000000000000000, 8.813324511995299047E-17 ) ) ;
#35807=ADVANCED_FACE ( 'NONE', ( #10982 ), #28211, .T. ) ;
#35811=EDGE_LOOP ( 'NONE', ( #3368, #11588, #2318, #19675 ) ) ;
#35842=CLOSED_SHELL ( 'NONE', ( #30823, #25016, #38873, #16413, #39693, #22107, #6551, #10871, #8686, #29764, #9603, #35807, #36847, #27075, #14089, #9981, #39937, #10208, #10370, #37118, #18654, #10060, #35714, #37246, #12673, #5115, #804, #23592, #40303, #5185, #31407, #30268, #28455, #31514, #9769, #15739, #21719, #25118, #42065, #42372, #21225, #1609, #4293, #23037, #38132, #32534, #28034, #13166, #23267, #9951, #15944, #34486, #29252, #32391, #21559, #24305, #40710, #5807, #26781 ) ) ;
#35959=DIRECTION ( 'NONE',  ( -1.000000000000000000, 3.469446951953614189E-17, 0.000000000000000000 ) ) ;
#35980=CARTESIAN_POINT ( 'NONE',  ( 22.90854556226730310, -34.05525454449573175, -74.83297477053802993 ) ) ;
#36007=FACE_OUTER_BOUND ( 'NONE', #31509, .T. ) ;
#36052=ORIENTED_EDGE ( 'NONE', *, *, #18500, .F. ) ;
#36068=DIRECTION ( 'NONE',  ( 3.009274222672345096E-17, 1.000000000000000000, -2.455023325076455345E-18 ) ) ;
#36144=CARTESIAN_POINT ( 'NONE',  ( 155.7547826636224499, -2.055254544495727309, 15.74958860255448734 ) ) ;
#36153=EDGE_CURVE ( 'NONE', #6816, #40515, #19455, .T. ) ;
#36160=EDGE_CURVE ( 'NONE', #6816, #9805, #16397, .T. ) ;
#36166=CIRCLE ( 'NONE', #18113, 11.00000000000000178 ) ;
#36179=CARTESIAN_POINT ( 'NONE',  ( -100.6569797752917879, -2.055254544495720648, -8.979913733870429127 ) ) ;
#36206=EDGE_CURVE ( 'NONE', #7972, #6816, #23629, .T. ) ;
#36252=CIRCLE ( 'NONE', #36289, 64.99999999999997158 ) ;
#36257=DIRECTION ( 'NONE',  ( 3.009274222672345096E-17, 1.000000000000000000, -2.455023325076454960E-18 ) ) ;
#36264=CARTESIAN_POINT ( 'NONE',  ( 42.80287614962723808, -34.05525454449571754, 69.29271901957299917 ) ) ;
#36269=CARTESIAN_POINT ( 'NONE',  ( -24.74979319748359785, 5.944745455504278020, 2.972870684497277427 ) ) ;
#36278=ORIENTED_EDGE ( 'NONE', *, *, #32005, .F. ) ;
#36283=FACE_OUTER_BOUND ( 'NONE', #24379, .T. ) ;
#36288=DIRECTION ( 'NONE',  ( 1.000000000000000000, 0.000000000000000000, 0.000000000000000000 ) ) ;
#36289=AXIS2_PLACEMENT_3D ( 'NONE', #43003, #26886, #36453 ) ;
#36388=DIRECTION ( 'NONE',  ( -3.009274222672345096E-17, -1.000000000000000000, 2.455023325076454960E-18 ) ) ;
#36406=FACE_OUTER_BOUND ( 'NONE', #26430, .T. ) ;
#36408=ORIENTED_EDGE ( 'NONE', *, *, #27058, .T. ) ;
#36424=ORIENTED_EDGE ( 'NONE', *, *, #29362, .F. ) ;
#36431=EDGE_LOOP ( 'NONE', ( #30780, #20562, #32777, #12193 ) ) ;
#36453=DIRECTION ( 'NONE',  ( -1.000000000000000000, 3.336006684570784581E-17, 0.000000000000000000 ) ) ;
#36463=DIRECTION ( 'NONE',  ( -1.000000000000000000, 1.084202172485505174E-16, 0.000000000000000000 ) ) ;
#36492=CIRCLE ( 'NONE', #39285, 10.99999999999999645 ) ;
#36504=AXIS2_PLACEMENT_3D ( 'NONE', #12150, #15860, #32629 ) ;
#36515=ORIENTED_EDGE ( 'NONE', *, *, #7103, .F. ) ;
#36522=ORIENTED_EDGE ( 'NONE', *, *, #14633, .T. ) ;
#36577=VERTEX_POINT ( 'NONE', #9932 ) ;
#36606=CARTESIAN_POINT ( 'NONE',  ( -8.749793197483594298, -2.055254544495723756, 2.972870684497274762 ) ) ;
#36613=AXIS2_PLACEMENT_3D ( 'NONE', #4847, #687, #17342 ) ;
#36629=VECTOR ( 'NONE', #5143, 1000.000000000000000 ) ;
#36650=DIRECTION ( 'NONE',  ( -1.000000000000000000, 2.668805347656626987E-17, 0.000000000000000000 ) ) ;
#36663=DIRECTION ( 'NONE',  ( 3.009274222672345096E-17, 1.000000000000000000, -2.455023325076455345E-18 ) ) ;
#36672=DIRECTION ( 'NONE',  ( 1.000000000000000000, 0.000000000000000000, 0.000000000000000000 ) ) ;
#36674=CARTESIAN_POINT ( 'NONE',  ( 26.80287614962791309, -12.05525454449571932, 69.29271901957253021 ) ) ;
#36692=DIRECTION ( 'NONE',  ( -1.000000000000000000, 2.668805347656626370E-17, 0.000000000000000000 ) ) ;
#36693=CIRCLE ( 'NONE', #41599, 10.49999999999998934 ) ;
#36738=DIRECTION ( 'NONE',  ( 1.000000000000000000, 0.000000000000000000, 0.000000000000000000 ) ) ;
#36847=ADVANCED_FACE ( 'NONE', ( #8822 ), #22387, .T. ) ;
#36861=LINE ( 'NONE', #30332, #14926 ) ;
#36868=ORIENTED_EDGE ( 'NONE', *, *, #20371, .T. ) ;
#36876=CARTESIAN_POINT ( 'NONE',  ( -8.749793197483594298, -12.05525454449572464, 2.972870684497274762 ) ) ;
#36930=ORIENTED_EDGE ( 'NONE', *, *, #17258, .T. ) ;
#36947=CARTESIAN_POINT ( 'NONE',  ( 12.40854556226731198, -34.05525454449573175, -74.83297477053802993 ) ) ;
#36953=EDGE_CURVE ( 'NONE', #4169, #11582, #6600, .T. ) ;
#36969=DIRECTION ( 'NONE',  ( -1.000000000000000000, 3.469446951953615421E-17, 0.000000000000000000 ) ) ;
#36993=AXIS2_PLACEMENT_3D ( 'NONE', #12768, #26074, #28924 ) ;
#37035=ORIENTED_EDGE ( 'NONE', *, *, #5601, .T. ) ;
#37041=ORIENTED_EDGE ( 'NONE', *, *, #10034, .T. ) ;
#37074=CARTESIAN_POINT ( 'NONE',  ( 11.90854556226686789, -14.05525454449572820, -74.83297477053821467 ) ) ;
#37118=ADVANCED_FACE ( 'NONE', ( #21268 ), #34745, .T. ) ;
#37157=EDGE_CURVE ( 'NONE', #42604, #11582, #25799, .T. ) ;
#37177=CIRCLE ( 'NONE', #7215, 10.49999999999999467 ) ;
#37188=DIRECTION ( 'NONE',  ( 1.058513553088275437E-16, 1.000000000000000000, -8.813324511995299047E-17 ) ) ;
#37196=AXIS2_PLACEMENT_3D ( 'NONE', #2349, #41663, #19013 ) ;
#37246=ADVANCED_FACE ( 'NONE', ( #36007 ), #29489, .F. ) ;
#37300=DIRECTION ( 'NONE',  ( -3.009274222672345096E-17, -1.000000000000000000, 2.455023325076454960E-18 ) ) ;
#37301=CIRCLE ( 'NONE', #39369, 15.99999999999998579 ) ;
#37338=FACE_OUTER_BOUND ( 'NONE', #26131, .T. ) ;
#37384=DIRECTION ( 'NONE',  ( -3.009274222672345096E-17, -1.000000000000000000, 2.455023325076454960E-18 ) ) ;
#37474=SURFACE_STYLE_USAGE ( .BOTH. , #27035 ) ;
#37479=DIRECTION ( 'NONE',  ( 1.058513553088275437E-16, 1.000000000000000000, -8.813324511995299047E-17 ) ) ;
#37480=EDGE_CURVE ( 'NONE', #19076, #37542, #23038, .T. ) ;
#37507=CARTESIAN_POINT ( 'NONE',  ( -23.34979319748359927, 5.944745455504278020, 2.972870684497277427 ) ) ;
#37509=DIRECTION ( 'NONE',  ( 1.058513553088275437E-16, 1.000000000000000000, -8.813324511995299047E-17 ) ) ;
#37529=DIRECTION ( 'NONE',  ( 3.009274222672345096E-17, 1.000000000000000000, -2.455023325076455345E-18 ) ) ;
#37542=VERTEX_POINT ( 'NONE', #29931 ) ;
#37750=EDGE_LOOP ( 'NONE', ( #36424, #39755, #9002, #18430 ) ) ;
#37782=PLANE ( 'NONE',  #13784 ) ;
#37818=DIRECTION ( 'NONE',  ( 3.009274222672345096E-17, 1.000000000000000000, -2.455023325076455345E-18 ) ) ;
#37865=ORIENTED_EDGE ( 'NONE', *, *, #13896, .F. ) ;
#37882=CARTESIAN_POINT ( 'NONE',  ( 33.90854556226734218, -14.05525454449573175, -74.83297477053821467 ) ) ;
#37898=FACE_OUTER_BOUND ( 'NONE', #27558, .T. ) ;
#37902=DIRECTION ( 'NONE',  ( 3.009274222672345096E-17, 1.000000000000000000, -2.455023325076455345E-18 ) ) ;
#37909=STYLED_ITEM ( 'NONE', ( #7589 ), #29166 ) ;
#37919=CARTESIAN_POINT ( 'NONE',  ( 47.90854556226721428, -2.055254544495724645, -74.83297477053847047 ) ) ;
#37926=VERTEX_POINT ( 'NONE', #26173 ) ;
#37961=DIRECTION ( 'NONE',  ( -3.009274222672345096E-17, -1.000000000000000000, 2.455023325076455345E-18 ) ) ;
#37971=CARTESIAN_POINT ( 'NONE',  ( -81.46080130434573618, -34.05525454449571043, 14.45886780445633946 ) ) ;
#37983=EDGE_CURVE ( 'NONE', #23828, #41341, #27159, .T. ) ;
#37998=VERTEX_POINT ( 'NONE', #16593 ) ;
#37999=EDGE_CURVE ( 'NONE', #28176, #39148, #32802, .T. ) ;
#38021=DIRECTION ( 'NONE',  ( -1.000000000000000000, 3.035766082959410566E-17, 0.000000000000000000 ) ) ;
#38047=LINE ( 'NONE', #42157, #40244 ) ;
#38050=DIRECTION ( 'NONE',  ( -1.058513553088275437E-16, -1.000000000000000000, 8.813324511995299047E-17 ) ) ;
#38092=CARTESIAN_POINT ( 'NONE',  ( 38.90854556226734218, -12.05525454449572997, -74.83297477053821467 ) ) ;
#38096=EDGE_CURVE ( 'NONE', #21731, #15816, #10416, .T. ) ;
#38121=DIRECTION ( 'NONE',  ( 3.009274222672345096E-17, 1.000000000000000000, -2.455023325076454960E-18 ) ) ;
#38132=ADVANCED_FACE ( 'NONE', ( #11315 ), #31168, .T. ) ;
#38143=CARTESIAN_POINT ( 'NONE',  ( 42.80287614962796994, -2.055254544495723756, 69.29271901957280022 ) ) ;
#38151=EDGE_CURVE ( 'NONE', #2586, #25188, #8424, .T. ) ;
#38204=CIRCLE ( 'NONE', #11774, 11.00000000000023803 ) ;
#38234=FACE_OUTER_BOUND ( 'NONE', #26823, .T. ) ;
#38270=VERTEX_POINT ( 'NONE', #2303 ) ;
#38303=ORIENTED_EDGE ( 'NONE', *, *, #982, .T. ) ;
#38326=DIRECTION ( 'NONE',  ( 1.000000000000000000, 0.000000000000000000, 0.000000000000000000 ) ) ;
#38328=DIRECTION ( 'NONE',  ( -1.000000000000000000, 0.000000000000000000, 0.000000000000000000 ) ) ;
#38329=EDGE_LOOP ( 'NONE', ( #4445, #24977, #39625, #28417 ) ) ;
#38421=VERTEX_POINT ( 'NONE', #42880 ) ;
#38453=ORIENTED_EDGE ( 'NONE', *, *, #21561, .T. ) ;
#38458=ORIENTED_EDGE ( 'NONE', *, *, #38096, .F. ) ;
#38468=ORIENTED_EDGE ( 'NONE', *, *, #25911, .T. ) ;
#38483=ORIENTED_EDGE ( 'NONE', *, *, #30198, .T. ) ;
#38489=AXIS2_PLACEMENT_3D ( 'NONE', #38769, #12189, #32871 ) ;
#38531=CARTESIAN_POINT ( 'NONE',  ( 53.80287614962789178, -40.05525454449572464, 69.29271901957253021 ) ) ;
#38590=ORIENTED_EDGE ( 'NONE', *, *, #27178, .F. ) ;
#38618=CARTESIAN_POINT ( 'NONE',  ( -107.9608013043457930, -12.05525454449572109, 14.45886780445738395 ) ) ;
#38643=EDGE_CURVE ( 'NONE', #4169, #9213, #20958, .T. ) ;
#38654=DIRECTION ( 'NONE',  ( 3.009274222672345096E-17, 1.000000000000000000, -2.455023325076454960E-18 ) ) ;
#38662=ORIENTED_EDGE ( 'NONE', *, *, #19639, .F. ) ;
#38698=CARTESIAN_POINT ( 'NONE',  ( -8.749793197483594298, -2.055254544495723756, 2.972870684497274762 ) ) ;
#38751=CARTESIAN_POINT ( 'NONE',  ( -36.79328511490363240, -12.05525454449572464, -55.66638716446937707 ) ) ;
#38769=CARTESIAN_POINT ( 'NONE',  ( 42.80287614962723808, -34.05525454449571754, 69.29271901957299917 ) ) ;
#38770=CARTESIAN_POINT ( 'NONE',  ( 6.908545562266867002, -12.05525454449572464, -74.83297477053821467 ) ) ;
#38776=AXIS2_PLACEMENT_3D ( 'NONE', #16716, #37384, #6853 ) ;
#38789=AXIS2_PLACEMENT_3D ( 'NONE', #15454, #12165, #1295 ) ;
#38792=VECTOR ( 'NONE', #4495, 1000.000000000000000 ) ;
#38797=AXIS2_PLACEMENT_3D ( 'NONE', #36606, #6727, #33560 ) ;
#38843=DIRECTION ( 'NONE',  ( -1.000000000000000000, 1.058513553088275437E-16, 0.000000000000000000 ) ) ;
#38873=ADVANCED_FACE ( 'NONE', ( #1931 ), #18572, .T. ) ;
#38881=EDGE_LOOP ( 'NONE', ( #3962, #38453 ) ) ;
#38936=DIRECTION ( 'NONE',  ( -1.000000000000000000, 0.000000000000000000, 0.000000000000000000 ) ) ;
#38969=CARTESIAN_POINT ( 'NONE',  ( -102.0670434220619427, -2.055254544495720648, 139.0496534599708980 ) ) ;
#38970=CARTESIAN_POINT ( 'NONE',  ( 2.339412683011424132, -12.05525454449572464, -89.04250581823735899 ) ) ;
#38992=PLANE ( 'NONE',  #22028 ) ;
#39015=FACE_OUTER_BOUND ( 'NONE', #28669, .T. ) ;
#39099=DIRECTION ( 'NONE',  ( -3.009274222672345096E-17, -1.000000000000000000, 2.455023325076454960E-18 ) ) ;
#39148=VERTEX_POINT ( 'NONE', #2728 ) ;
#39156=ORIENTED_EDGE ( 'NONE', *, *, #4012, .T. ) ;
#39162=VERTEX_POINT ( 'NONE', #29389 ) ;
#39171=DIRECTION ( 'NONE',  ( -1.000000000000000000, 0.000000000000000000, 0.000000000000000000 ) ) ;
#39183=CARTESIAN_POINT ( 'NONE',  ( -102.9608013043458072, -14.05525454449570688, 14.45886780445738218 ) ) ;
#39198=AXIS2_PLACEMENT_3D ( 'NONE', #22235, #42018, #16295 ) ;
#39285=AXIS2_PLACEMENT_3D ( 'NONE', #11829, #4826, #18619 ) ;
#39325=EDGE_LOOP ( 'NONE', ( #35512, #22108 ) ) ;
#39331=ORIENTED_EDGE ( 'NONE', *, *, #27184, .T. ) ;
#39339=CYLINDRICAL_SURFACE ( 'NONE', #36993, 100.0000000000000000 ) ;
#39355=CARTESIAN_POINT ( 'NONE',  ( 42.80287614962790599, -34.05525454449571754, 69.29271901957253021 ) ) ;
#39369=AXIS2_PLACEMENT_3D ( 'NONE', #23699, #10360, #4002 ) ;
#39374=CARTESIAN_POINT ( 'NONE',  ( -19.74979319748359430, 117.9447454555042754, 2.972870684497276539 ) ) ;
#39403=AXIS2_PLACEMENT_3D ( 'NONE', #26504, #19987, #19129 ) ;
#39406=ORIENTED_EDGE ( 'NONE', *, *, #3906, .T. ) ;
#39450=ORIENTED_EDGE ( 'NONE', *, *, #10034, .F. ) ;
#39492=AXIS2_PLACEMENT_3D ( 'NONE', #28626, #21470, #35359 ) ;
#39493=CARTESIAN_POINT ( 'NONE',  ( -36.94957890273524725, -2.055254544495720648, 165.5452302238048503 ) ) ;
#39532=DIRECTION ( 'NONE',  ( -3.009274222672345096E-17, -1.000000000000000000, 2.455023325076454960E-18 ) ) ;
#39548=ORIENTED_EDGE ( 'NONE', *, *, #14324, .F. ) ;
#39625=ORIENTED_EDGE ( 'NONE', *, *, #3936, .T. ) ;
#39693=ADVANCED_FACE ( 'NONE', ( #36283 ), #6401, .T. ) ;
#39705=CARTESIAN_POINT ( 'NONE',  ( 22.90854556226710415, -34.05525454449573175, -74.83297477053821467 ) ) ;
#39731=VERTEX_POINT ( 'NONE', #40846 ) ;
#39755=ORIENTED_EDGE ( 'NONE', *, *, #15315, .F. ) ;
#39793=CARTESIAN_POINT ( 'NONE',  ( 32.30287614962725229, -35.35525454449572180, 69.29271901957299917 ) ) ;
#39797=CIRCLE ( 'NONE', #6360, 24.99999999999998934 ) ;
#39855=CARTESIAN_POINT ( 'NONE',  ( 2.339412683011424576, -2.055254544495723756, -89.04250581823735899 ) ) ;
#39869=CARTESIAN_POINT ( 'NONE',  ( -91.96080130434580724, -34.05525454449571043, 14.45886780445738218 ) ) ;
#39880=EDGE_LOOP ( 'NONE', ( #30422, #15099 ) ) ;
#39884=SHAPE_DEFINITION_REPRESENTATION ( #6402, #10434 ) ;
#39888=EDGE_CURVE ( 'NONE', #1360, #2343, #16162, .T. ) ;
#39914=DIRECTION ( 'NONE',  ( 3.009274222672345096E-17, 1.000000000000000000, -2.455023325076454960E-18 ) ) ;
#39937=ADVANCED_FACE ( 'NONE', ( #8137 ), #18221, .T. ) ;
#39987=CARTESIAN_POINT ( 'NONE',  ( 56.05503971749756431, -2.055254544495723756, 8.006123197671259462 ) ) ;
#40040=VECTOR ( 'NONE', #6885, 1000.000000000000000 ) ;
#40055=DIRECTION ( 'NONE',  ( 3.009274222672345096E-17, 1.000000000000000000, -2.455023325076454960E-18 ) ) ;
#40066=CIRCLE ( 'NONE', #14330, 25.00000000000002132 ) ;
#40085=CARTESIAN_POINT ( 'NONE',  ( 146.1418929693599580, -12.05525454449572820, -53.89157828313137344 ) ) ;
#40111=CARTESIAN_POINT ( 'NONE',  ( -102.4608013043457362, -34.05525454449571043, 14.45886780445633946 ) ) ;
#40112=EDGE_CURVE ( 'NONE', #40515, #12272, #2406, .T. ) ;
#40155=ORIENTED_EDGE ( 'NONE', *, *, #4159, .T. ) ;
#40174=CARTESIAN_POINT ( 'NONE',  ( 31.80287614962791665, -14.05525454449571754, 69.29271901957253021 ) ) ;
#40244=VECTOR ( 'NONE', #35421, 1000.000000000000000 ) ;
#40272=DIRECTION ( 'NONE',  ( -1.000000000000000000, 0.000000000000000000, 0.000000000000000000 ) ) ;
#40303=ADVANCED_FACE ( 'NONE', ( #23192 ), #20145, .T. ) ;
#40344=EDGE_LOOP ( 'NONE', ( #36515, #6555, #5695, #3720 ) ) ;
#40429=DIRECTION ( 'NONE',  ( -3.009274222672345096E-17, -1.000000000000000000, 2.455023325076454960E-18 ) ) ;
#40433=AXIS2_PLACEMENT_3D ( 'NONE', #12879, #6954, #29675 ) ;
#40448=AXIS2_PLACEMENT_3D ( 'NONE', #10884, #31381, #4085 ) ;
#40476=AXIS2_PLACEMENT_3D ( 'NONE', #12494, #28649, #32322 ) ;
#40515=VERTEX_POINT ( 'NONE', #5867 ) ;
#40530=FACE_OUTER_BOUND ( 'NONE', #22529, .T. ) ;
#40563=LINE ( 'NONE', #21439, #3692 ) ;
#40592=CYLINDRICAL_SURFACE ( 'NONE', #42242, 11.00000000000023448 ) ;
#40602=CARTESIAN_POINT ( 'NONE',  ( -8.749793197483594298, -12.05525454449572464, 2.972870684497274762 ) ) ;
#40610=EDGE_LOOP ( 'NONE', ( #6547, #15554, #40832, #36522 ) ) ;
#40612=ORIENTED_EDGE ( 'NONE', *, *, #42792, .T. ) ;
#40615=DIRECTION ( 'NONE',  ( 3.009274222672345096E-17, 1.000000000000000000, -2.455023325076455345E-18 ) ) ;
#40639=DIRECTION ( 'NONE',  ( -3.009274222672345096E-17, -1.000000000000000000, 2.455023325076454960E-18 ) ) ;
#40667=CARTESIAN_POINT ( 'NONE',  ( 47.55521504368574881, -2.055254544495723756, -70.64469547305695585 ) ) ;
#40681=ORIENTED_EDGE ( 'NONE', *, *, #7567, .T. ) ;
#40708=CIRCLE ( 'NONE', #21968, 15.99999999999998934 ) ;
#40710=ADVANCED_FACE ( 'NONE', ( #19866 ), #33135, .T. ) ;
#40716=CARTESIAN_POINT ( 'NONE',  ( 33.90854556226734218, -35.35525454449573601, -74.83297477053821467 ) ) ;
#40746=CARTESIAN_POINT ( 'NONE',  ( 22.90854556226710415, -14.05525454449572997, -74.83297477053821467 ) ) ;
#40776=COLOUR_RGB ( '', 0.66274510, 0.83137255, 0.94901961) ;
#40815=CIRCLE ( 'NONE', #36613, 100.0000000000000000 ) ;
#40818=LINE ( 'NONE', #43077, #26889 ) ;
#40820=EDGE_LOOP ( 'NONE', ( #13138, #2489 ) ) ;
#40832=ORIENTED_EDGE ( 'NONE', *, *, #36206, .F. ) ;
#40846=CARTESIAN_POINT ( 'NONE',  ( 26.85238513915532721, -12.05525454449572464, 88.54322126041917329 ) ) ;
#40873=CIRCLE ( 'NONE', #38797, 64.99999999999998579 ) ;
#40898=DIRECTION ( 'NONE',  ( -1.058513553088275437E-16, -1.000000000000000000, 8.813324511995299047E-17 ) ) ;
#40922=CARTESIAN_POINT ( 'NONE',  ( 42.80287614962790599, -40.05525454449572464, 69.29271901957253021 ) ) ;
#41032=EDGE_CURVE ( 'NONE', #18808, #11152, #39797, .T. ) ;
#41044=CARTESIAN_POINT ( 'NONE',  ( 22.90854556226722138, -2.055254544495723756, -74.83297477053847047 ) ) ;
#41047=CARTESIAN_POINT ( 'NONE',  ( -8.749793197483592522, 117.9447454555042754, 2.972870684497274762 ) ) ;
#41050=ORIENTED_EDGE ( 'NONE', *, *, #17048, .T. ) ;
#41183=FACE_OUTER_BOUND ( 'NONE', #775, .T. ) ;
#41209=ORIENTED_EDGE ( 'NONE', *, *, #1684, .F. ) ;
#41225=FACE_OUTER_BOUND ( 'NONE', #25181, .T. ) ;
#41273=DIRECTION ( 'NONE',  ( -1.000000000000000000, 3.336006684570784581E-17, 0.000000000000000000 ) ) ;
#41284=CARTESIAN_POINT ( 'NONE',  ( -36.94957890273524725, -2.055254544495720648, 165.5452302238048503 ) ) ;
#41341=VERTEX_POINT ( 'NONE', #8560 ) ;
#41376=AXIS2_PLACEMENT_3D ( 'NONE', #15703, #29430, #19204 ) ;
#41380=CARTESIAN_POINT ( 'NONE',  ( -91.96080130434580724, -12.05525454449572109, 14.45886780445738218 ) ) ;
#41383=CARTESIAN_POINT ( 'NONE',  ( 67.80287614962797704, -12.05525454449572464, 69.29271901957280022 ) ) ;
#41411=CARTESIAN_POINT ( 'NONE',  ( -97.01392236320388918, -2.055254544495720648, 76.75426063221412676 ) ) ;
#41430=CIRCLE ( 'NONE', #9355, 100.0000000000000000 ) ;
#41437=CIRCLE ( 'NONE', #30994, 100.0000000000000000 ) ;
#41440=EDGE_LOOP ( 'NONE', ( #20203, #523, #36868, #17274 ) ) ;
#41456=VERTEX_POINT ( 'NONE', #18867 ) ;
#41463=VECTOR ( 'NONE', #13816, 1000.000000000000000 ) ;
#41491=AXIS2_PLACEMENT_3D ( 'NONE', #24930, #7430, #646 ) ;
#41535=AXIS2_PLACEMENT_3D ( 'NONE', #41411, #41849, #34880 ) ;
#41590=EDGE_LOOP ( 'NONE', ( #9848, #20963, #33699, #28996 ) ) ;
#41599=AXIS2_PLACEMENT_3D ( 'NONE', #24954, #27991, #8745 ) ;
#41608=DIRECTION ( 'NONE',  ( -3.009274222672345096E-17, -1.000000000000000000, 2.455023325076454960E-18 ) ) ;
#41632=CIRCLE ( 'NONE', #15875, 100.0000000000000000 ) ;
#41663=DIRECTION ( 'NONE',  ( -3.009274222672345096E-17, -1.000000000000000000, 2.455023325076454960E-18 ) ) ;
#41684=ORIENTED_EDGE ( 'NONE', *, *, #42315, .T. ) ;
#41689=VERTEX_POINT ( 'NONE', #33409 ) ;
#41694=CIRCLE ( 'NONE', #30567, 11.00000000000000178 ) ;
#41848=ORIENTED_EDGE ( 'NONE', *, *, #20882, .F. ) ;
#41849=DIRECTION ( 'NONE',  ( 3.009274222672345096E-17, 1.000000000000000000, -2.455023325076454960E-18 ) ) ;
#41904=VERTEX_POINT ( 'NONE', #22719 ) ;
#42009=ORIENTED_EDGE ( 'NONE', *, *, #39888, .T. ) ;
#42018=DIRECTION ( 'NONE',  ( -3.009274222672345712E-17, -1.000000000000000000, 2.455023325076455345E-18 ) ) ;
#42022=LINE ( 'NONE', #18115, #28305 ) ;
#42065=ADVANCED_FACE ( 'NONE', ( #40530, #26613 ), #610, .F. ) ;
#42066=EDGE_CURVE ( 'NONE', #17546, #18529, #27055, .T. ) ;
#42094=CARTESIAN_POINT ( 'NONE',  ( 22.90854556226710415, -14.05525454449572997, -74.83297477053821467 ) ) ;
#42157=CARTESIAN_POINT ( 'NONE',  ( -102.4608013043457362, -35.35525454449571470, 14.45886780445633946 ) ) ;
#42171=ORIENTED_EDGE ( 'NONE', *, *, #2772, .T. ) ;
#42190=CYLINDRICAL_SURFACE ( 'NONE', #25887, 99.99999999999994316 ) ;
#42223=DIRECTION ( 'NONE',  ( 1.000000000000000000, 0.000000000000000000, 0.000000000000000000 ) ) ;
#42229=DIRECTION ( 'NONE',  ( 3.009274222672345096E-17, 1.000000000000000000, -2.455023325076454960E-18 ) ) ;
#42242=AXIS2_PLACEMENT_3D ( 'NONE', #7451, #671, #30808 ) ;
#42258=AXIS2_PLACEMENT_3D ( 'NONE', #12360, #12777, #38936 ) ;
#42299=CARTESIAN_POINT ( 'NONE',  ( -107.9608013043457930, -14.05525454449570866, 14.45886780445738395 ) ) ;
#42315=EDGE_CURVE ( 'NONE', #25188, #2586, #26686, .T. ) ;
#42348=DIRECTION ( 'NONE',  ( -1.000000000000000000, 3.469446951953614189E-17, 0.000000000000000000 ) ) ;
#42372=ADVANCED_FACE ( 'NONE', ( #28571 ), #8677, .T. ) ;
#42390=VECTOR ( 'NONE', #19901, 1000.000000000000000 ) ;
#42398=DIRECTION ( 'NONE',  ( -3.009274222672345096E-17, -1.000000000000000000, 2.455023325076455345E-18 ) ) ;
#42441=EDGE_LOOP ( 'NONE', ( #23574, #15729 ) ) ;
#42446=VERTEX_POINT ( 'NONE', #26357 ) ;
#42506=FACE_OUTER_BOUND ( 'NONE', #34454, .T. ) ;
#42568=EDGE_LOOP ( 'NONE', ( #18513, #29776 ) ) ;
#42599=CYLINDRICAL_SURFACE ( 'NONE', #20066, 1.399999999999998579 ) ;
#42604=VERTEX_POINT ( 'NONE', #27868 ) ;
#42617=VERTEX_POINT ( 'NONE', #24171 ) ;
#42692=DIRECTION ( 'NONE',  ( 1.000000000000000000, -1.058513553088275437E-16, 0.000000000000000000 ) ) ;
#42725=DIRECTION ( 'NONE',  ( -3.009274222672345096E-17, -1.000000000000000000, 2.455023325076454960E-18 ) ) ;
#42762=EDGE_CURVE ( 'NONE', #39148, #28176, #21926, .T. ) ;
#42776=DIRECTION ( 'NONE',  ( -1.000000000000000000, 3.469446951953611107E-17, 0.000000000000000000 ) ) ;
#42788=AXIS2_PLACEMENT_3D ( 'NONE', #25398, #38654, #16869 ) ;
#42792=EDGE_CURVE ( 'NONE', #36577, #13563, #31986, .T. ) ;
#42815=ORIENTED_EDGE ( 'NONE', *, *, #21746, .F. ) ;
#42861=( GEOMETRIC_REPRESENTATION_CONTEXT ( 3 ) GLOBAL_UNCERTAINTY_ASSIGNED_CONTEXT ( ( #24378 ) ) GLOBAL_UNIT_ASSIGNED_CONTEXT ( ( #17378, #13438, #27170 ) ) REPRESENTATION_CONTEXT ( 'NONE', 'WORKASPACE' ) );
#42880=CARTESIAN_POINT ( 'NONE',  ( -81.46080130434573618, -35.35525454449571470, 14.45886780445633946 ) ) ;
#42956=EDGE_CURVE ( 'NONE', #5150, #17494, #27531, .T. ) ;
#43003=CARTESIAN_POINT ( 'NONE',  ( -8.749793197483594298, -2.055254544495723756, 2.972870684497274762 ) ) ;
#43023=ORIENTED_EDGE ( 'NONE', *, *, #43033, .T. ) ;
#43031=DIRECTION ( 'NONE',  ( 1.000000000000000000, -3.336006684570783348E-17, 0.000000000000000000 ) ) ;
#43033=EDGE_CURVE ( 'NONE', #2987, #33446, #36492, .T. ) ;
#43036=EDGE_LOOP ( 'NONE', ( #19409, #12513, #39406, #16856 ) ) ;
#43077=CARTESIAN_POINT ( 'NONE',  ( 2.250206802516407034, 117.9447454555042754, 2.972870684497274762 ) ) ;
#43083=EDGE_CURVE ( 'NONE', #19640, #14319, #10768, .T. ) ;
#43096=ORIENTED_EDGE ( 'NONE', *, *, #11522, .F. ) ;
#43113=VERTEX_POINT ( 'NONE', #37971 ) ;
#43148=ORIENTED_EDGE ( 'NONE', *, *, #27314, .T. ) ;
#43163=AXIS2_PLACEMENT_3D ( 'NONE', #7906, #27563, #10991 ) ;
#43182=CARTESIAN_POINT ( 'NONE',  ( -91.96080130434580724, -35.35525454449571470, 14.45886780445738218 ) ) ;
ENDSEC;
END-ISO-10303-21;
